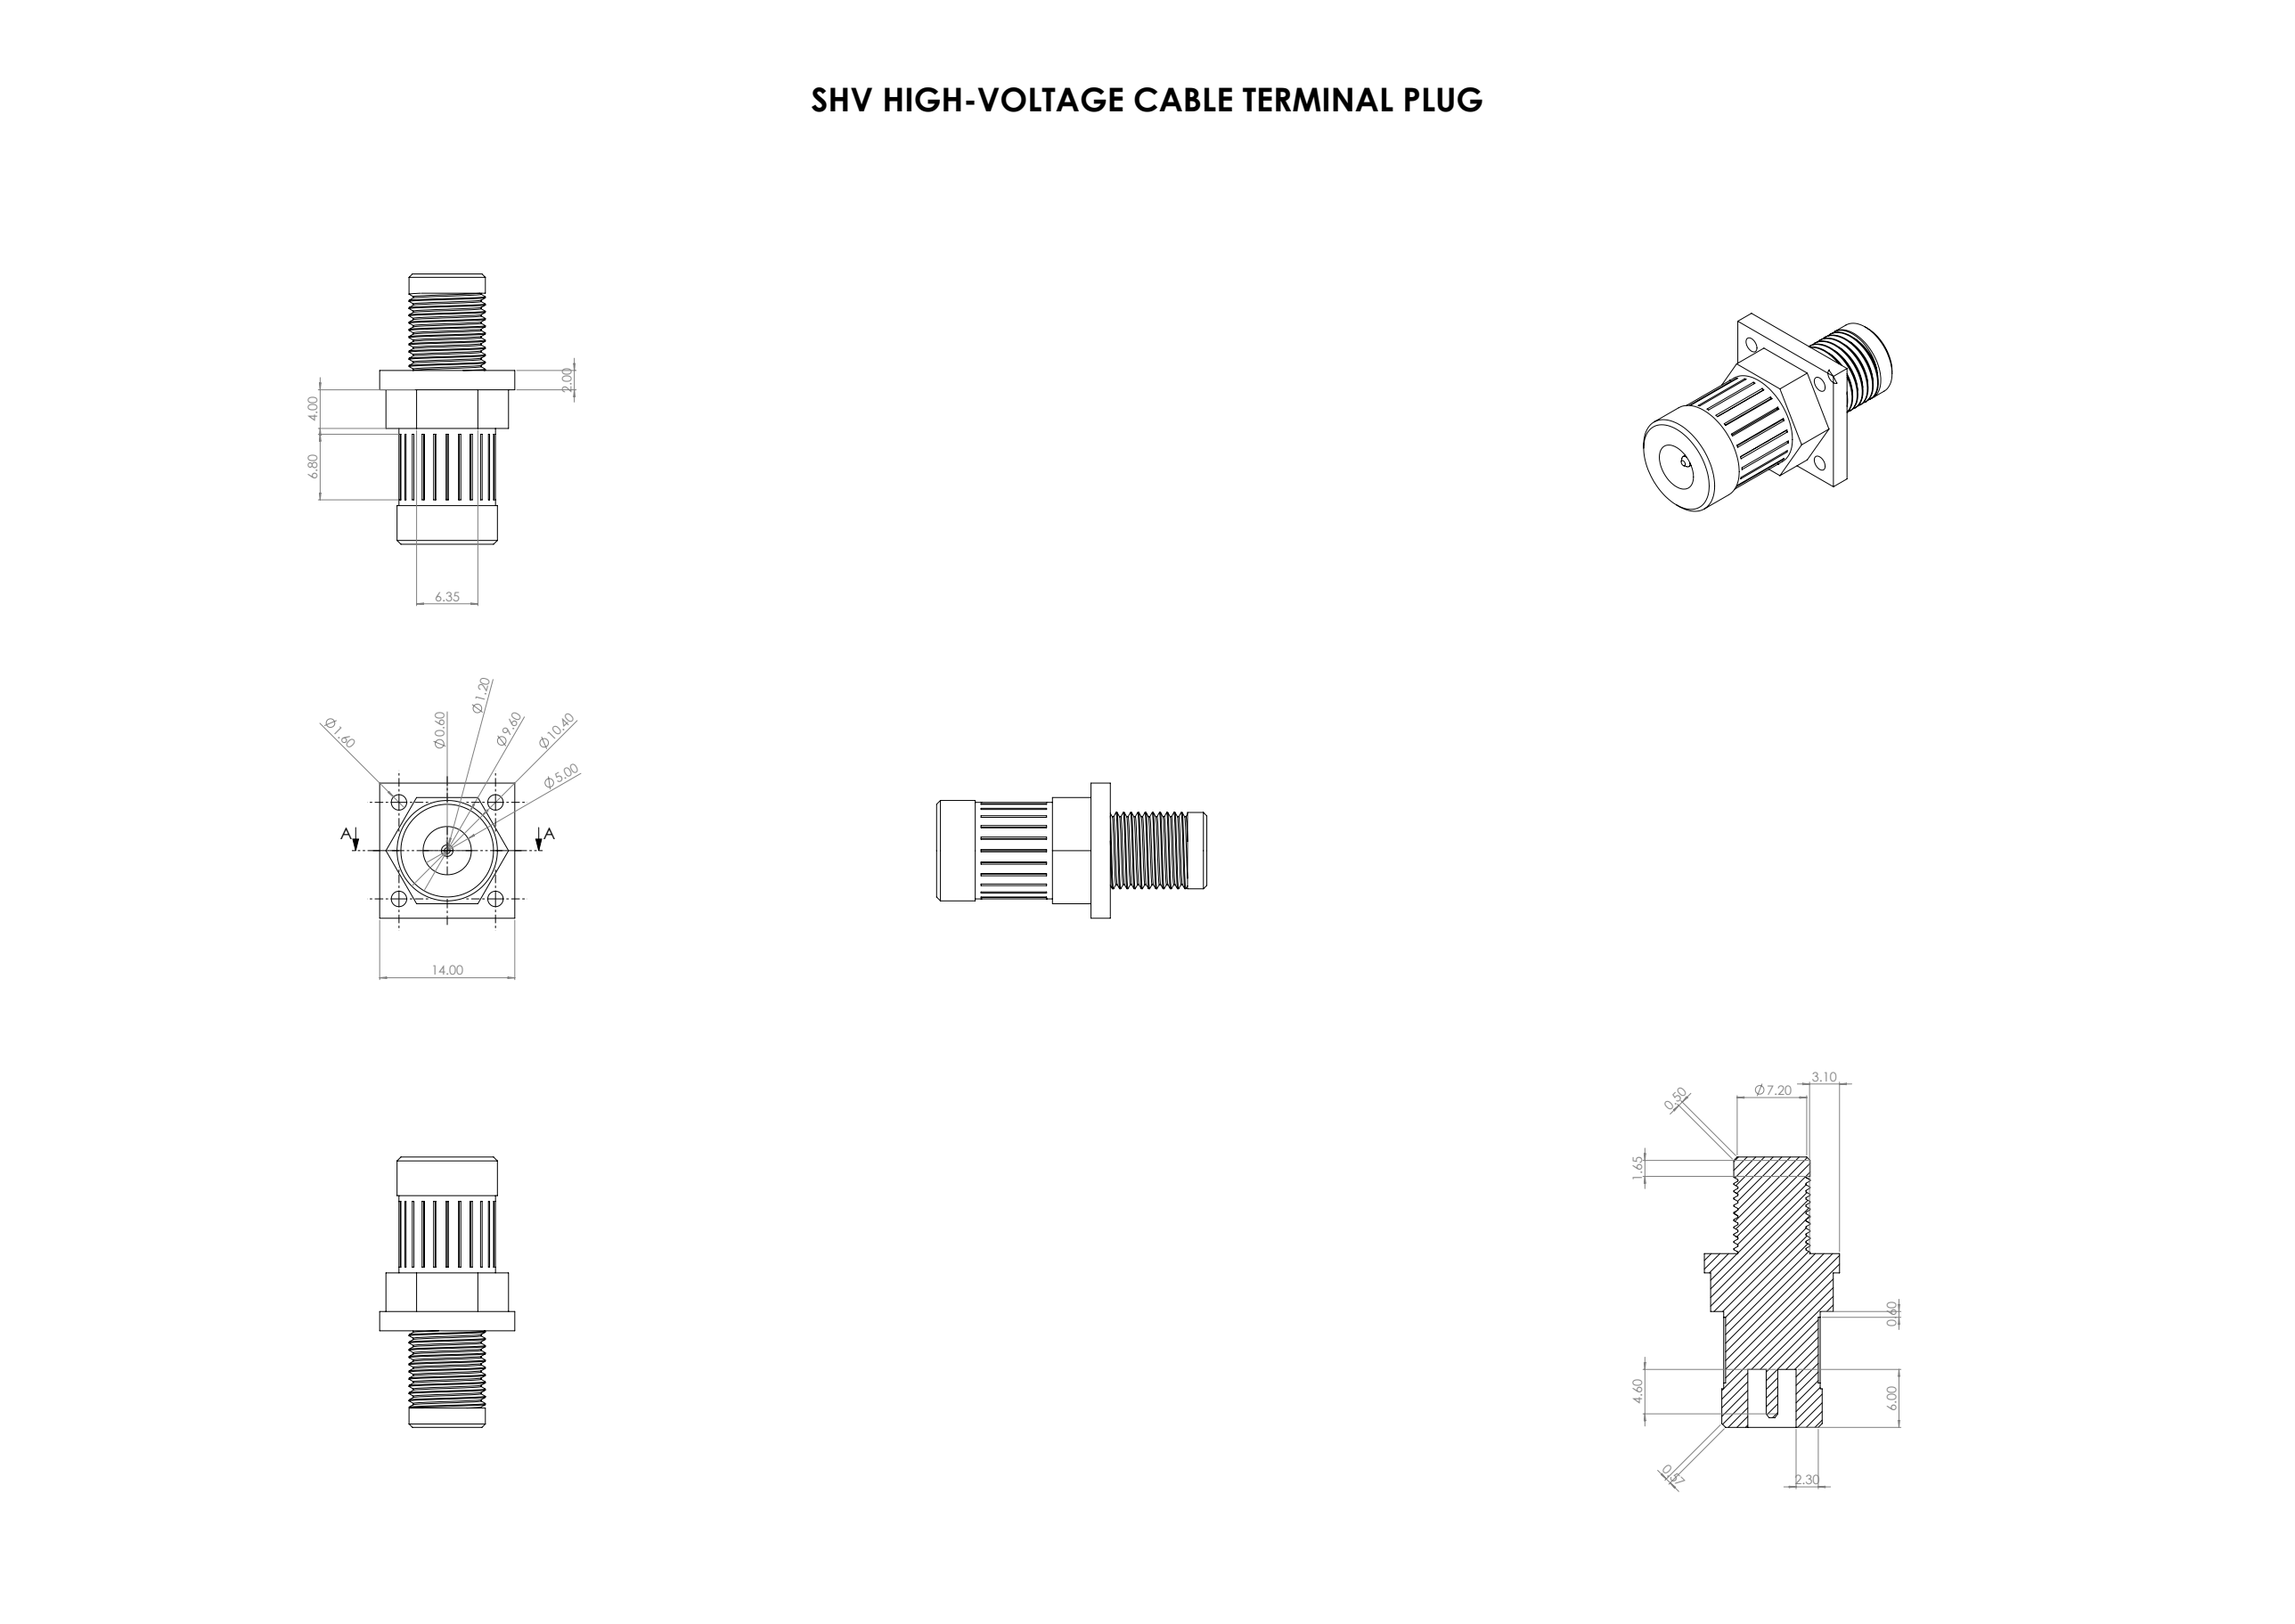
ISO-10303-21;
HEADER;
/* Generated by software containing ST-Developer
 * from STEP Tools, Inc. (www.steptools.com) 
 */

FILE_DESCRIPTION(
/* description */ (''),
/* implementation_level */ '2;1');

FILE_NAME(
/* name */ '13_SHV_High-Voltage_Cable_Terminal_Plug.step',
/* time_stamp */ '2026-10-19T22:59:19-07:00',
/* author */ (''),
/* organization */ (''),
/* preprocessor_version */ 'ST-DEVELOPER v20.2',
/* originating_system */ 'Autodesk Translation Framework v15.15.0.0',
/* authorisation */ '');

FILE_SCHEMA (('AUTOMOTIVE_DESIGN { 1 0 10303 214 3 1 1 }'));
ENDSEC;

DATA;
#10=MECHANICAL_DESIGN_GEOMETRIC_PRESENTATION_REPRESENTATION('',(#916),#53650);
#363=B_SPLINE_SURFACE_WITH_KNOTS('',3,3,((#34003,#34004,#34005,#34006,#34007,
#34008,#34009,#34010,#34011,#34012,#34013,#34014,#34015,#34016,#34017,#34018,
#34019,#34020,#34021,#34022,#34023,#34024,#34025,#34026,#34027,#34028,#34029,
#34030,#34031,#34032,#34033,#34034,#34035,#34036,#34037,#34038,#34039,#34040,
#34041,#34042,#34043,#34044,#34045,#34046,#34047,#34048,#34049,#34050,#34051,
#34052,#34053,#34054,#34055,#34056,#34057,#34058,#34059,#34060,#34061,#34062,
#34063,#34064,#34065,#34066,#34067,#34068,#34069,#34070,#34071,#34072,#34073,
#34074,#34075),(#34076,#34077,#34078,#34079,#34080,#34081,#34082,#34083,
#34084,#34085,#34086,#34087,#34088,#34089,#34090,#34091,#34092,#34093,#34094,
#34095,#34096,#34097,#34098,#34099,#34100,#34101,#34102,#34103,#34104,#34105,
#34106,#34107,#34108,#34109,#34110,#34111,#34112,#34113,#34114,#34115,#34116,
#34117,#34118,#34119,#34120,#34121,#34122,#34123,#34124,#34125,#34126,#34127,
#34128,#34129,#34130,#34131,#34132,#34133,#34134,#34135,#34136,#34137,#34138,
#34139,#34140,#34141,#34142,#34143,#34144,#34145,#34146,#34147,#34148),
(#34149,#34150,#34151,#34152,#34153,#34154,#34155,#34156,#34157,#34158,
#34159,#34160,#34161,#34162,#34163,#34164,#34165,#34166,#34167,#34168,#34169,
#34170,#34171,#34172,#34173,#34174,#34175,#34176,#34177,#34178,#34179,#34180,
#34181,#34182,#34183,#34184,#34185,#34186,#34187,#34188,#34189,#34190,#34191,
#34192,#34193,#34194,#34195,#34196,#34197,#34198,#34199,#34200,#34201,#34202,
#34203,#34204,#34205,#34206,#34207,#34208,#34209,#34210,#34211,#34212,#34213,
#34214,#34215,#34216,#34217,#34218,#34219,#34220,#34221),(#34222,#34223,
#34224,#34225,#34226,#34227,#34228,#34229,#34230,#34231,#34232,#34233,#34234,
#34235,#34236,#34237,#34238,#34239,#34240,#34241,#34242,#34243,#34244,#34245,
#34246,#34247,#34248,#34249,#34250,#34251,#34252,#34253,#34254,#34255,#34256,
#34257,#34258,#34259,#34260,#34261,#34262,#34263,#34264,#34265,#34266,#34267,
#34268,#34269,#34270,#34271,#34272,#34273,#34274,#34275,#34276,#34277,#34278,
#34279,#34280,#34281,#34282,#34283,#34284,#34285,#34286,#34287,#34288,#34289,
#34290,#34291,#34292,#34293,#34294)),.UNSPECIFIED.,.F.,.F.,.F.,(4,4),(4,
1,1,1,1,1,1,1,1,1,1,1,1,1,1,1,1,1,1,1,1,1,1,1,1,1,1,1,1,1,1,1,1,1,1,1,1,
1,1,1,1,1,1,1,1,1,1,1,1,1,1,1,1,1,1,1,1,1,1,1,1,1,1,1,1,1,1,1,1,1,4),(0.,
0.0496809906637673),(9.51827045652186,10.5054372529097,11.4926040492975,
12.4797708456853,13.4669376420731,14.4541044384609,15.4412712348487,16.4284380312366,
17.4156048276244,18.4027716240122,19.3899384204,20.3771052167878,21.3642720131756,
22.3514388095634,23.3386056059513,24.3257724023391,25.3129391987269,26.3001059951147,
27.2872727915025,28.2744395878903,29.2616063842781,30.2487731806659,31.2359399770538,
32.2231067734416,33.2102735698294,34.1974403662172,35.184607162605,36.1717739589928,
37.1589407553806,38.1461075517685,39.1332743481563,40.1204411445441,41.1076079409319,
42.0947747373197,43.0819415337075,44.0691083300953,45.0562751264832,46.043441922871,
47.0306087192588,48.0177755156466,49.0049423120344,49.9921091084222,50.97927590481,
51.9664427011978,52.9536094975857,53.9407762939735,54.9279430903613,55.9151098867491,
56.9022766831369,57.8894434795247,58.8766102759126,59.8637770723004,60.8509438686882,
61.838110665076,62.8252774614638,63.8124442578516,64.7996110542394,65.7867778506272,
66.7739446470151,67.7611114434029,68.7482782397907,69.7354450361785,70.7226118325663,
71.7097786289541,72.696945425342,73.6841122217298,74.6712790181176,75.6584458145054,
76.6456126108932,77.632779407281,78.6199462036688),.UNSPECIFIED.);
#364=B_SPLINE_SURFACE_WITH_KNOTS('',3,3,((#34517,#34518,#34519,#34520,#34521,
#34522,#34523,#34524,#34525,#34526,#34527,#34528,#34529,#34530,#34531,#34532,
#34533,#34534,#34535,#34536,#34537,#34538,#34539,#34540,#34541,#34542,#34543,
#34544,#34545,#34546,#34547,#34548,#34549,#34550,#34551,#34552,#34553,#34554,
#34555,#34556,#34557,#34558,#34559,#34560,#34561,#34562,#34563,#34564,#34565,
#34566,#34567,#34568,#34569,#34570,#34571,#34572,#34573,#34574,#34575,#34576,
#34577,#34578,#34579,#34580,#34581,#34582,#34583,#34584,#34585,#34586,#34587,
#34588,#34589),(#34590,#34591,#34592,#34593,#34594,#34595,#34596,#34597,
#34598,#34599,#34600,#34601,#34602,#34603,#34604,#34605,#34606,#34607,#34608,
#34609,#34610,#34611,#34612,#34613,#34614,#34615,#34616,#34617,#34618,#34619,
#34620,#34621,#34622,#34623,#34624,#34625,#34626,#34627,#34628,#34629,#34630,
#34631,#34632,#34633,#34634,#34635,#34636,#34637,#34638,#34639,#34640,#34641,
#34642,#34643,#34644,#34645,#34646,#34647,#34648,#34649,#34650,#34651,#34652,
#34653,#34654,#34655,#34656,#34657,#34658,#34659,#34660,#34661,#34662),
(#34663,#34664,#34665,#34666,#34667,#34668,#34669,#34670,#34671,#34672,
#34673,#34674,#34675,#34676,#34677,#34678,#34679,#34680,#34681,#34682,#34683,
#34684,#34685,#34686,#34687,#34688,#34689,#34690,#34691,#34692,#34693,#34694,
#34695,#34696,#34697,#34698,#34699,#34700,#34701,#34702,#34703,#34704,#34705,
#34706,#34707,#34708,#34709,#34710,#34711,#34712,#34713,#34714,#34715,#34716,
#34717,#34718,#34719,#34720,#34721,#34722,#34723,#34724,#34725,#34726,#34727,
#34728,#34729,#34730,#34731,#34732,#34733,#34734,#34735),(#34736,#34737,
#34738,#34739,#34740,#34741,#34742,#34743,#34744,#34745,#34746,#34747,#34748,
#34749,#34750,#34751,#34752,#34753,#34754,#34755,#34756,#34757,#34758,#34759,
#34760,#34761,#34762,#34763,#34764,#34765,#34766,#34767,#34768,#34769,#34770,
#34771,#34772,#34773,#34774,#34775,#34776,#34777,#34778,#34779,#34780,#34781,
#34782,#34783,#34784,#34785,#34786,#34787,#34788,#34789,#34790,#34791,#34792,
#34793,#34794,#34795,#34796,#34797,#34798,#34799,#34800,#34801,#34802,#34803,
#34804,#34805,#34806,#34807,#34808)),.UNSPECIFIED.,.F.,.F.,.F.,(4,4),(4,
1,1,1,1,1,1,1,1,1,1,1,1,1,1,1,1,1,1,1,1,1,1,1,1,1,1,1,1,1,1,1,1,1,1,1,1,
1,1,1,1,1,1,1,1,1,1,1,1,1,1,1,1,1,1,1,1,1,1,1,1,1,1,1,1,1,1,1,1,1,4),(0.,
0.0496809906637673),(12.8380991276371,13.8252659240249,14.8124327204127,
15.7995995168005,16.7867663131883,17.7739331095761,18.7610999059639,19.7482667023518,
20.7354334987396,21.7226002951274,22.7097670915152,23.696933887903,24.6841006842908,
25.6712674806786,26.6584342770665,27.6456010734543,28.6327678698421,29.6199346662299,
30.6071014626177,31.5942682590055,32.5814350553933,33.5686018517812,34.555768648169,
35.5429354445568,36.5301022409446,37.5172690373324,38.5044358337202,39.491602630108,
40.4787694264959,41.4659362228837,42.4531030192715,43.4402698156593,44.4274366120471,
45.4146034084349,46.4017702048227,47.3889370012105,48.3761037975984,49.3632705939862,
50.350437390374,51.3376041867618,52.3247709831496,53.3119377795374,54.2991045759252,
55.2862713723131,56.2734381687009,57.2606049650887,58.2477717614765,59.2349385578643,
60.2221053542521,61.2092721506399,62.1964389470278,63.1836057434156,64.1707725398034,
65.1579393361912,66.145106132579,67.1322729289668,68.1194397253546,69.1066065217424,
70.0937733181303,71.0809401145181,72.0681069109059,73.0552737072937,74.0424405036815,
75.0296073000693,76.0167740964572,77.003940892845,77.9911076892328,78.9782744856206,
79.9654412820084,80.9526080783962,81.939774874784),.UNSPECIFIED.);
#373=B_SPLINE_CURVE_WITH_KNOTS('',3,(#33239,#33240,#33241,#33242,#33243,
#33244,#33245,#33246,#33247,#33248,#33249,#33250,#33251,#33252,#33253,#33254,
#33255,#33256,#33257,#33258,#33259,#33260,#33261,#33262,#33263),
 .UNSPECIFIED.,.F.,.F.,(4,3,3,3,3,3,3,3,4),(-9.15304944749145,-8.88450116749033,
-7.89733437110252,-6.9101675747147,-5.92300077832689,-4.93583398193907,
-3.94866718555126,-2.96150038916344,-2.86986414031186),.UNSPECIFIED.);
#374=B_SPLINE_CURVE_WITH_KNOTS('',3,(#33268,#33269,#33270,#33271),
 .UNSPECIFIED.,.F.,.F.,(4,4),(-2.86986414031186,-2.08103247056473),
 .UNSPECIFIED.);
#375=B_SPLINE_CURVE_WITH_KNOTS('',3,(#33274,#33275,#33276,#33277,#33278,
#33279,#33280,#33281,#33282,#33283,#33284,#33285,#33286,#33287,#33288,#33289,
#33290,#33291,#33292,#33293,#33294,#33295),.UNSPECIFIED.,.F.,.F.,(4,3,3,
3,3,3,3,4),(0.,0.98716679638781,1.97433359277563,2.96150038916344,3.94866718555125,
4.93583398193907,5.92300077832688,6.18969281142703),.UNSPECIFIED.);
#376=B_SPLINE_CURVE_WITH_KNOTS('',3,(#33300,#33301,#33302,#33303,#33304,
#33305,#33306,#33307,#33308,#33309,#33310,#33311,#33312,#33313,#33314,#33315,
#33316,#33317,#33318,#33319,#33320,#33321),.UNSPECIFIED.,.F.,.F.,(4,3,3,
3,3,3,3,4),(-15.436234754671,-14.8075019458172,-13.8203351494294,-12.8331683530416,
-11.8460015566538,-10.858834760266,-9.87166796387814,-9.15304944749145),
 .UNSPECIFIED.);
#377=B_SPLINE_CURVE_WITH_KNOTS('',3,(#33322,#33323,#33324,#33325,#33326,
#33327,#33328,#33329,#33330,#33331,#33332,#33333,#33334,#33335,#33336,#33337,
#33338,#33339,#33340,#33341,#33342,#33343),.UNSPECIFIED.,.F.,.F.,(4,3,3,
3,3,3,3,4),(6.18969281142703,6.9101675747147,7.89733437110251,8.88450116749032,
9.87166796387814,10.858834760266,11.8460015566538,12.4728781186066),
 .UNSPECIFIED.);
#378=B_SPLINE_CURVE_WITH_KNOTS('',3,(#33348,#33349,#33350,#33351,#33352,
#33353,#33354,#33355,#33356,#33357,#33358,#33359,#33360,#33361,#33362,#33363,
#33364,#33365,#33366,#33367,#33368,#33369),.UNSPECIFIED.,.F.,.F.,(4,3,3,
3,3,3,3,4),(-21.7194200618506,-20.7305027241441,-19.7433359277563,-18.7561691313685,
-17.7690023349807,-16.7818355385928,-15.794668742205,-15.436234754671),
 .UNSPECIFIED.);
#379=B_SPLINE_CURVE_WITH_KNOTS('',3,(#33370,#33371,#33372,#33373,#33374,
#33375,#33376,#33377,#33378,#33379,#33380,#33381,#33382,#33383,#33384,#33385,
#33386,#33387,#33388,#33389,#33390,#33391),.UNSPECIFIED.,.F.,.F.,(4,3,3,
3,3,3,3,4),(12.4728781186066,12.8331683530416,13.8203351494294,14.8075019458172,
15.794668742205,16.7818355385928,17.7690023349807,18.7560634257862),
 .UNSPECIFIED.);
#380=B_SPLINE_CURVE_WITH_KNOTS('',3,(#33396,#33397,#33398,#33399,#33400,
#33401,#33402,#33403,#33404,#33405,#33406,#33407,#33408,#33409,#33410,#33411,
#33412,#33413,#33414,#33415,#33416,#33417),.UNSPECIFIED.,.F.,.F.,(4,3,3,
3,3,3,3,4),(-28.0026053690302,-27.6406702988588,-26.653503502471,-25.6663367060832,
-24.6791699096953,-23.6920031133075,-22.7048363169197,-21.7194200618506),
 .UNSPECIFIED.);
#381=B_SPLINE_CURVE_WITH_KNOTS('',3,(#33418,#33419,#33420,#33421,#33422,
#33423,#33424,#33425,#33426,#33427,#33428,#33429,#33430,#33431,#33432,#33433,
#33434,#33435,#33436,#33437,#33438,#33439),.UNSPECIFIED.,.F.,.F.,(4,3,3,
3,3,3,3,4),(18.7560634257862,19.7433359277563,20.7305027241441,21.7176695205319,
22.7048363169197,23.6920031133075,24.6791699096954,25.0392487329658),
 .UNSPECIFIED.);
#382=B_SPLINE_CURVE_WITH_KNOTS('',3,(#33444,#33445,#33446,#33447,#33448,
#33449,#33450,#33451,#33452,#33453,#33454,#33455,#33456,#33457,#33458,#33459,
#33460,#33461,#33462,#33463,#33464,#33465),.UNSPECIFIED.,.F.,.F.,(4,3,3,
3,3,3,3,4),(-34.2857906762098,-33.5636710771857,-32.5765042807979,-31.58933748441,
-30.6021706880222,-29.6150038916344,-28.6278370952466,-28.0026053690302),
 .UNSPECIFIED.);
#383=B_SPLINE_CURVE_WITH_KNOTS('',3,(#33466,#33467,#33468,#33469,#33470,
#33471,#33472,#33473,#33474,#33475,#33476,#33477,#33478,#33479,#33480,#33481,
#33482,#33483,#33484,#33485,#33486,#33487),.UNSPECIFIED.,.F.,.F.,(4,3,3,
3,3,3,3,4),(25.0392487329658,25.6663367060832,26.653503502471,27.6406702988588,
28.6278370952466,29.6150038916344,30.6021706880222,31.3224340401454),
 .UNSPECIFIED.);
#384=B_SPLINE_CURVE_WITH_KNOTS('',3,(#33492,#33493,#33494,#33495,#33496,
#33497,#33498,#33499,#33500,#33501,#33502,#33503,#33504,#33505,#33506,#33507,
#33508,#33509,#33510,#33511,#33512,#33513,#33514,#33515,#33516),
 .UNSPECIFIED.,.F.,.F.,(4,3,3,3,3,3,3,3,4),(-40.5689759833894,-40.4738386519004,
-39.4866718555126,-38.4995050591247,-37.5123382627369,-36.5251714663491,
-35.5380046699613,-34.5508378735735,-34.2857906762098),.UNSPECIFIED.);
#385=B_SPLINE_CURVE_WITH_KNOTS('',3,(#33517,#33518,#33519,#33520,#33521,
#33522,#33523,#33524,#33525,#33526,#33527,#33528,#33529,#33530,#33531,#33532,
#33533,#33534,#33535,#33536,#33537,#33538,#33539,#33540,#33541),
 .UNSPECIFIED.,.F.,.F.,(4,3,3,3,3,3,3,3,4),(31.3224340401454,31.58933748441,
32.5765042807979,33.5636710771857,34.5508378735735,35.5380046699613,36.5251714663491,
37.5123382627369,37.605619347325),.UNSPECIFIED.);
#386=B_SPLINE_CURVE_WITH_KNOTS('',3,(#33546,#33547,#33548,#33549,#33550,
#33551,#33552,#33553,#33554,#33555,#33556,#33557,#33558,#33559,#33560,#33561,
#33562,#33563,#33564,#33565,#33566,#33567),.UNSPECIFIED.,.F.,.F.,(4,3,3,
3,3,3,3,4),(-46.852161290569,-46.3968394302273,-45.4096726338394,-44.4225058374516,
-43.4353390410638,-42.448172244676,-41.4610054482882,-40.5689759833894),
 .UNSPECIFIED.);
#387=B_SPLINE_CURVE_WITH_KNOTS('',3,(#33568,#33569,#33570,#33571,#33572,
#33573,#33574,#33575,#33576,#33577,#33578,#33579,#33580,#33581,#33582,#33583,
#33584,#33585,#33586,#33587,#33588,#33589),.UNSPECIFIED.,.F.,.F.,(4,3,3,
3,3,3,3,4),(37.605619347325,38.4995050591248,39.4866718555126,40.4738386519004,
41.4610054482882,42.448172244676,43.4353390410638,43.8888046545046),
 .UNSPECIFIED.);
#388=B_SPLINE_CURVE_WITH_KNOTS('',3,(#33594,#33595,#33596,#33597,#33598,
#33599,#33600,#33601,#33602,#33603,#33604,#33605,#33606,#33607,#33608,#33609,
#33610,#33611,#33612,#33613,#33614,#33615),.UNSPECIFIED.,.F.,.F.,(4,3,3,
3,3,3,3,4),(-53.1353465977486,-52.3198402085541,-51.3326734121663,-50.3455066157785,
-49.3583398193907,-48.3711730230029,-47.3840062266151,-46.852161290569),
 .UNSPECIFIED.);
#389=B_SPLINE_CURVE_WITH_KNOTS('',3,(#33616,#33617,#33618,#33619,#33620,
#33621,#33622,#33623,#33624,#33625,#33626,#33627,#33628,#33629,#33630,#33631,
#33632,#33633,#33634,#33635,#33636,#33637),.UNSPECIFIED.,.F.,.F.,(4,3,3,
3,3,3,3,4),(43.8888046545046,44.4225058374516,45.4096726338394,46.3968394302273,
47.3840062266151,48.3711730230029,49.3583398193907,50.1719899616841),
 .UNSPECIFIED.);
#390=B_SPLINE_CURVE_WITH_KNOTS('',3,(#33642,#33643,#33644,#33645,#33646,
#33647,#33648,#33649,#33650,#33651,#33652,#33653,#33654,#33655,#33656,#33657,
#33658,#33659,#33660,#33661,#33662,#33663,#33664,#33665,#33666),
 .UNSPECIFIED.,.F.,.F.,(4,3,3,3,3,3,3,3,4),(-59.4185319049282,-59.2300077832689,
-58.242840986881,-57.2556741904932,-56.2685073941054,-55.2813405977176,
-54.2941738013298,-53.307007004942,-53.1353465977486),.UNSPECIFIED.);
#391=B_SPLINE_CURVE_WITH_KNOTS('',3,(#33667,#33668,#33669,#33670,#33671,
#33672,#33673,#33674,#33675,#33676,#33677,#33678,#33679,#33680,#33681,#33682,
#33683,#33684,#33685,#33686,#33687,#33688,#33689,#33690,#33691),
 .UNSPECIFIED.,.F.,.F.,(4,3,3,3,3,3,3,3,4),(50.1719899616841,50.3455066157785,
51.3326734121663,52.3198402085541,53.307007004942,54.2941738013298,55.2813405977176,
56.2685073941054,56.4551752688637),.UNSPECIFIED.);
#392=B_SPLINE_CURVE_WITH_KNOTS('',3,(#33696,#33697,#33698,#33699,#33700,
#33701,#33702,#33703,#33704,#33705,#33706,#33707,#33708,#33709,#33710,#33711,
#33712,#33713,#33714,#33715,#33716,#33717),.UNSPECIFIED.,.F.,.F.,(4,3,3,
3,3,3,3,4),(-65.7017172121077,-65.1530085615957,-64.1658417652079,-63.1786749688201,
-62.1915081724323,-61.2043413760445,-60.2171745796567,-59.4185319049282),
 .UNSPECIFIED.);
#393=B_SPLINE_CURVE_WITH_KNOTS('',3,(#33718,#33719,#33720,#33721,#33722,
#33723,#33724,#33725,#33726,#33727,#33728,#33729,#33730,#33731,#33732,#33733,
#33734,#33735,#33736,#33737,#33738,#33739),.UNSPECIFIED.,.F.,.F.,(4,3,3,
3,3,3,3,4),(56.4551752688637,57.2556741904932,58.242840986881,59.2300077832688,
60.2171745796566,61.2043413760445,62.1915081724323,62.7383605760433),
 .UNSPECIFIED.);
#394=B_SPLINE_CURVE_WITH_KNOTS('',3,(#33745,#33746,#33747,#33748,#33749),
 .UNSPECIFIED.,.F.,.F.,(4,1,4),(78.5398163397448,78.9782744856206,79.8587424042193),
 .UNSPECIFIED.);
#395=B_SPLINE_CURVE_WITH_KNOTS('',3,(#33752,#33753,#33754,#33755),
 .UNSPECIFIED.,.F.,.F.,(4,4),(78.5398163397448,78.6199462036688),
 .UNSPECIFIED.);
#396=B_SPLINE_CURVE_WITH_KNOTS('',3,(#33760,#33761,#33762,#33763,#33764,
#33765,#33766,#33767,#33768,#33769),.UNSPECIFIED.,.F.,.F.,(4,1,1,1,1,1,
1,4),(72.2566310325652,73.0552737072937,74.0424405036815,75.0296073000693,
76.0167740964572,77.003940892845,77.9911076892328,78.5398163397448),
 .UNSPECIFIED.);
#397=B_SPLINE_CURVE_WITH_KNOTS('',3,(#33770,#33771,#33772,#33773,#33774,
#33775,#33776,#33777,#33778,#33779),.UNSPECIFIED.,.F.,.F.,(4,1,1,1,1,1,
1,4),(72.2566310325652,72.696945425342,73.6841122217298,74.6712790181176,
75.6584458145054,76.6456126108932,77.632779407281,78.5398163397448),
 .UNSPECIFIED.);
#398=B_SPLINE_CURVE_WITH_KNOTS('',3,(#33784,#33785,#33786,#33787,#33788,
#33789,#33790,#33791,#33792,#33793,#33794),.UNSPECIFIED.,.F.,.F.,(4,1,1,
1,1,1,1,1,4),(65.9734457253856,66.145106132579,67.1322729289668,68.1194397253546,
69.1066065217424,70.0937733181303,71.0809401145181,72.0681069109059,72.2566310325652),
 .UNSPECIFIED.);
#399=B_SPLINE_CURVE_WITH_KNOTS('',3,(#33795,#33796,#33797,#33798,#33799,
#33800,#33801,#33802,#33803,#33804),.UNSPECIFIED.,.F.,.F.,(4,1,1,1,1,1,
1,4),(65.9734457253856,66.7739446470151,67.7611114434029,68.7482782397907,
69.7354450361785,70.7226118325663,71.7097786289541,72.2566310325652),
 .UNSPECIFIED.);
#400=B_SPLINE_CURVE_WITH_KNOTS('',3,(#33809,#33810,#33811,#33812,#33813,
#33814,#33815,#33816,#33817,#33818),.UNSPECIFIED.,.F.,.F.,(4,1,1,1,1,1,
1,4),(59.6902604182061,60.2221053542521,61.2092721506399,62.1964389470278,
63.1836057434156,64.1707725398034,65.1579393361912,65.9734457253856),
 .UNSPECIFIED.);
#401=B_SPLINE_CURVE_WITH_KNOTS('',3,(#33819,#33820,#33821,#33822,#33823,
#33824,#33825,#33826,#33827,#33828,#33829),.UNSPECIFIED.,.F.,.F.,(4,1,1,
1,1,1,1,1,4),(59.6902604182061,59.8637770723004,60.8509438686882,61.838110665076,
62.8252774614638,63.8124442578516,64.7996110542394,65.7867778506272,65.9734457253856),
 .UNSPECIFIED.);
#402=B_SPLINE_CURVE_WITH_KNOTS('',3,(#33834,#33835,#33836,#33837,#33838,
#33839,#33840,#33841,#33842,#33843),.UNSPECIFIED.,.F.,.F.,(4,1,1,1,1,1,
1,4),(53.4070751110265,54.2991045759252,55.2862713723131,56.2734381687009,
57.2606049650887,58.2477717614765,59.2349385578643,59.6902604182061),
 .UNSPECIFIED.);
#403=B_SPLINE_CURVE_WITH_KNOTS('',3,(#33844,#33845,#33846,#33847,#33848,
#33849,#33850,#33851,#33852,#33853),.UNSPECIFIED.,.F.,.F.,(4,1,1,1,1,1,
1,4),(53.4070751110265,53.9407762939735,54.9279430903613,55.9151098867491,
56.9022766831369,57.8894434795247,58.8766102759126,59.6902604182061),
 .UNSPECIFIED.);
#404=B_SPLINE_CURVE_WITH_KNOTS('',3,(#33858,#33859,#33860,#33861,#33862,
#33863,#33864,#33865,#33866,#33867,#33868),.UNSPECIFIED.,.F.,.F.,(4,1,1,
1,1,1,1,1,4),(47.1238898038469,47.3889370012105,48.3761037975984,49.3632705939862,
50.350437390374,51.3376041867618,52.3247709831496,53.3119377795374,53.4070751110265),
 .UNSPECIFIED.);
#405=B_SPLINE_CURVE_WITH_KNOTS('',3,(#33869,#33870,#33871,#33872,#33873,
#33874,#33875,#33876,#33877,#33878),.UNSPECIFIED.,.F.,.F.,(4,1,1,1,1,1,
1,4),(47.1238898038469,48.0177755156466,49.0049423120344,49.9921091084222,
50.97927590481,51.9664427011978,52.9536094975857,53.4070751110265),
 .UNSPECIFIED.);
#406=B_SPLINE_CURVE_WITH_KNOTS('',3,(#33883,#33884,#33885,#33886,#33887,
#33888,#33889,#33890,#33891,#33892),.UNSPECIFIED.,.F.,.F.,(4,1,1,1,1,1,
1,4),(40.8407044966673,41.4659362228837,42.4531030192715,43.4402698156593,
44.4274366120471,45.4146034084349,46.4017702048227,47.1238898038469),
 .UNSPECIFIED.);
#407=B_SPLINE_CURVE_WITH_KNOTS('',3,(#33893,#33894,#33895,#33896,#33897,
#33898,#33899,#33900,#33901,#33902,#33903),.UNSPECIFIED.,.F.,.F.,(4,1,1,
1,1,1,1,1,4),(40.8407044966673,41.1076079409319,42.0947747373197,43.0819415337075,
44.0691083300953,45.0562751264832,46.043441922871,47.0306087192588,47.1238898038469),
 .UNSPECIFIED.);
#408=B_SPLINE_CURVE_WITH_KNOTS('',3,(#33908,#33909,#33910,#33911,#33912,
#33913,#33914,#33915,#33916,#33917),.UNSPECIFIED.,.F.,.F.,(4,1,1,1,1,1,
1,4),(34.5575191894877,35.5429354445568,36.5301022409446,37.5172690373324,
38.5044358337202,39.491602630108,40.4787694264959,40.8407044966673),
 .UNSPECIFIED.);
#409=B_SPLINE_CURVE_WITH_KNOTS('',3,(#33918,#33919,#33920,#33921,#33922,
#33923,#33924,#33925,#33926,#33927),.UNSPECIFIED.,.F.,.F.,(4,1,1,1,1,1,
1,4),(34.5575191894877,35.184607162605,36.1717739589928,37.1589407553806,
38.1461075517685,39.1332743481563,40.1204411445441,40.8407044966673),
 .UNSPECIFIED.);
#410=B_SPLINE_CURVE_WITH_KNOTS('',3,(#33932,#33933,#33934,#33935,#33936,
#33937,#33938,#33939,#33940,#33941,#33942),.UNSPECIFIED.,.F.,.F.,(4,1,1,
1,1,1,1,1,4),(28.2743338823081,28.6327678698421,29.6199346662299,30.6071014626177,
31.5942682590055,32.5814350553933,33.5686018517812,34.555768648169,34.5575191894877),
 .UNSPECIFIED.);
#411=B_SPLINE_CURVE_WITH_KNOTS('',3,(#33943,#33944,#33945,#33946,#33947,
#33948,#33949,#33950,#33951,#33952,#33953),.UNSPECIFIED.,.F.,.F.,(4,1,1,
1,1,1,1,1,4),(28.2743338823081,28.2744395878903,29.2616063842781,30.2487731806659,
31.2359399770538,32.2231067734416,33.2102735698294,34.1974403662172,34.5575191894877),
 .UNSPECIFIED.);
#412=B_SPLINE_CURVE_WITH_KNOTS('',3,(#33958,#33959,#33960,#33961,#33962,
#33963,#33964,#33965,#33966,#33967),.UNSPECIFIED.,.F.,.F.,(4,1,1,1,1,1,
1,4),(21.9911485751285,22.7097670915152,23.696933887903,24.6841006842908,
25.6712674806786,26.6584342770665,27.6456010734543,28.2743338823081),
 .UNSPECIFIED.);
#413=B_SPLINE_CURVE_WITH_KNOTS('',3,(#33968,#33969,#33970,#33971,#33972,
#33973,#33974,#33975,#33976,#33977),.UNSPECIFIED.,.F.,.F.,(4,1,1,1,1,1,
1,4),(21.9911485751285,22.3514388095634,23.3386056059513,24.3257724023391,
25.3129391987269,26.3001059951147,27.2872727915025,28.2743338823081),
 .UNSPECIFIED.);
#414=B_SPLINE_CURVE_WITH_KNOTS('',3,(#33982,#33983,#33984,#33985,#33986,
#33987,#33988,#33989,#33990,#33991,#33992),.UNSPECIFIED.,.F.,.F.,(4,1,1,
1,1,1,1,1,4),(15.7079632679489,15.7995995168005,16.7867663131883,17.7739331095761,
18.7610999059639,19.7482667023518,20.7354334987396,21.7226002951274,21.9911485751285),
 .UNSPECIFIED.);
#415=B_SPLINE_CURVE_WITH_KNOTS('',3,(#33993,#33994,#33995,#33996,#33997,
#33998,#33999,#34000,#34001,#34002),.UNSPECIFIED.,.F.,.F.,(4,1,1,1,1,1,
1,4),(15.7079632679489,16.4284380312366,17.4156048276244,18.4027716240122,
19.3899384204,20.3771052167878,21.3642720131756,21.9911485751285),
 .UNSPECIFIED.);
#416=B_SPLINE_CURVE_WITH_KNOTS('',3,(#34296,#34297,#34298,#34299,#34300,
#34301,#34302,#34303,#34304,#34305,#34306,#34307,#34308,#34309,#34310,#34311,
#34312,#34313,#34314,#34315,#34316,#34317,#34318,#34319,#34320,#34321,#34322,
#34323,#34324,#34325,#34326,#34327,#34328,#34329,#34330,#34331,#34332,#34333,
#34334,#34335,#34336,#34337,#34338,#34339,#34340,#34341,#34342,#34343,#34344,
#34345,#34346,#34347,#34348,#34349,#34350,#34351,#34352,#34353,#34354,#34355,
#34356),.UNSPECIFIED.,.F.,.F.,(4,3,3,3,3,3,3,3,3,3,3,3,3,3,3,3,3,3,3,3,
4),(-0.780432929098612,-0.738338012777856,-0.683834258573259,-0.663838565476387,
-0.598169338795401,-0.577510604236597,-0.562119826273733,-0.497408932506566,
-0.451782302166264,-0.430327346583771,-0.415002532446257,-0.359442543267042,
-0.314512225358661,-0.29120578257896,-0.270249996878916,-0.207616527572625,
-0.155712395679469,-0.140396343062156,-0.123829552848863,-0.0619147764244314,
0.),.UNSPECIFIED.);
#417=B_SPLINE_CURVE_WITH_KNOTS('',3,(#34357,#34358,#34359,#34360,#34361,
#34362,#34363,#34364,#34365,#34366,#34367,#34368,#34369,#34370,#34371,#34372),
 .UNSPECIFIED.,.F.,.F.,(4,3,3,3,3,4),(62.7383605760433,63.1786749688201,
64.1658417652079,65.1530085615957,66.1401753579835,67.0206432765822),
 .UNSPECIFIED.);
#418=B_SPLINE_CURVE_WITH_KNOTS('',3,(#34374,#34375,#34376,#34377,#34378,
#34379,#34380,#34381,#34382,#34383,#34384,#34385,#34386,#34387,#34388,#34389,
#34390,#34391,#34392,#34393,#34394,#34395,#34396,#34397,#34398,#34399,#34400,
#34401,#34402,#34403,#34404,#34405,#34406,#34407,#34408,#34409,#34410,#34411,
#34412,#34413,#34414,#34415,#34416,#34417,#34418,#34419,#34420,#34421,#34422,
#34423,#34424,#34425,#34426,#34427,#34428,#34429,#34430,#34431,#34432,#34433,
#34434,#34435,#34436,#34437),.UNSPECIFIED.,.F.,.F.,(4,3,3,3,3,3,3,3,3,3,
3,3,3,3,3,3,3,3,3,3,3,4),(-0.782320427274649,-0.744412510134687,-0.688529792301629,
-0.669642910660232,-0.618424444943536,-0.597739729117171,-0.580869545572353,
-0.517475334412603,-0.472408188284826,-0.451438075940233,-0.43660958913821,
-0.382241417220766,-0.33446124006817,-0.310889038365519,-0.29130300268306,
-0.227103495746363,-0.170327621809772,-0.152876921934579,-0.137524083313296,
-0.0687620416566481,-0.00415757966036404,0.),.UNSPECIFIED.);
#419=B_SPLINE_CURVE_WITH_KNOTS('',3,(#34438,#34439,#34440,#34441,#34442,
#34443,#34444,#34445),.UNSPECIFIED.,.F.,.F.,(4,1,1,1,1,4),(11.5993029270866,
12.4797708456853,13.4669376420731,14.4541044384609,15.4412712348487,15.7079632679489),
 .UNSPECIFIED.);
#420=B_SPLINE_CURVE_WITH_KNOTS('',3,(#34448,#34449,#34450,#34451,#34452,
#34453,#34454,#34455,#34456,#34457,#34458,#34459,#34460,#34461,#34462,#34463,
#34464,#34465,#34466,#34467,#34468,#34469,#34470,#34471,#34472,#34473,#34474,
#34475,#34476,#34477,#34478,#34479,#34480,#34481,#34482,#34483,#34484,#34485,
#34486,#34487,#34488,#34489,#34490,#34491,#34492,#34493,#34494,#34495,#34496,
#34497,#34498,#34499,#34500,#34501,#34502,#34503,#34504,#34505,#34506,#34507,
#34508),.UNSPECIFIED.,.F.,.F.,(4,3,3,3,3,3,3,3,3,3,3,3,3,3,3,3,3,3,3,3,
4),(-0.780432929098611,-0.738338012777859,-0.683834237462397,-0.663838555047122,
-0.598169328522835,-0.577510488075,-0.562119617951329,-0.497408718040529,
-0.45178193717698,-0.430324802159164,-0.415000406365485,-0.359442543267047,
-0.314512225358666,-0.29120578372101,-0.27024999961834,-0.207616508984274,
-0.155712381738205,-0.140396296964378,-0.123829546509967,-0.0619147732549836,
0.),.UNSPECIFIED.);
#421=B_SPLINE_CURVE_WITH_KNOTS('',3,(#34511,#34512,#34513,#34514,#34515,
#34516),.UNSPECIFIED.,.F.,.F.,(4,1,1,4),(12.8380991276371,13.8252659240249,
14.8124327204127,15.7079632679489),.UNSPECIFIED.);
#422=B_SPLINE_CURVE_WITH_KNOTS('',3,(#34810,#34811,#34812,#34813,#34814,
#34815,#34816,#34817,#34818,#34819,#34820,#34821,#34822,#34823,#34824,#34825,
#34826,#34827,#34828,#34829,#34830,#34831,#34832,#34833,#34834,#34835,#34836,
#34837,#34838,#34839,#34840,#34841,#34842,#34843,#34844,#34845,#34846,#34847,
#34848,#34849,#34850,#34851,#34852,#34853,#34854,#34855,#34856,#34857,#34858,
#34859,#34860,#34861,#34862,#34863,#34864,#34865,#34866,#34867,#34868,#34869,
#34870,#34871,#34872,#34873),.UNSPECIFIED.,.F.,.F.,(4,3,3,3,3,3,3,3,3,3,
3,3,3,3,3,3,3,3,3,3,3,4),(-0.782320427274647,-0.744412510134681,-0.688529784827506,
-0.669642900569953,-0.618424486060736,-0.597739627606828,-0.580869476506375,
-0.5174752643267,-0.472408127669552,-0.451437419639239,-0.436608276654843,
-0.38224141722077,-0.334461240068174,-0.310889049141467,-0.291303007297222,
-0.227103471436237,-0.170327603577178,-0.152876814667526,-0.137524066743929,
-0.0687620333719644,-0.00415763970634024,0.),.UNSPECIFIED.);
#423=B_SPLINE_CURVE_WITH_KNOTS('',3,(#34874,#34875,#34876,#34877,#34878,
#34879,#34880,#34881,#34882,#34883,#34884,#34885,#34886),.UNSPECIFIED.,
 .F.,.F.,(4,3,3,3,4),(-69.101675747147,-68.1145089507592,-67.1273421543714,
-66.1401753579836,-65.7017172121077),.UNSPECIFIED.);
#884=SHAPE_REPRESENTATION_RELATIONSHIP('SRR','None',#53729,#900);
#900=ADVANCED_BREP_SHAPE_REPRESENTATION('',(#932),#53639);
#916=STYLED_ITEM('',(#53972),#932);
#932=MANIFOLD_SOLID_BREP('SHV Plug',#23308);
#1000=CYLINDRICAL_SURFACE('',#24108,0.3954);
#1001=CYLINDRICAL_SURFACE('',#24111,0.3954);
#1002=CYLINDRICAL_SURFACE('',#24112,0.3954);
#1003=CYLINDRICAL_SURFACE('',#24113,0.3954);
#1004=CYLINDRICAL_SURFACE('',#24114,0.3954);
#1005=CYLINDRICAL_SURFACE('',#24115,0.3954);
#1006=CYLINDRICAL_SURFACE('',#24116,0.3954);
#1007=CYLINDRICAL_SURFACE('',#24117,0.3954);
#1008=CYLINDRICAL_SURFACE('',#24118,0.3954);
#1009=CYLINDRICAL_SURFACE('',#24119,0.3954);
#1010=CYLINDRICAL_SURFACE('',#24120,0.352375);
#1011=CYLINDRICAL_SURFACE('',#24122,0.352375);
#1012=CYLINDRICAL_SURFACE('',#24123,0.352375);
#1013=CYLINDRICAL_SURFACE('',#24124,0.352375);
#1014=CYLINDRICAL_SURFACE('',#24125,0.352375);
#1015=CYLINDRICAL_SURFACE('',#24126,0.352375);
#1016=CYLINDRICAL_SURFACE('',#24127,0.352375);
#1017=CYLINDRICAL_SURFACE('',#24128,0.352375);
#1018=CYLINDRICAL_SURFACE('',#24129,0.352375);
#1019=CYLINDRICAL_SURFACE('',#24130,0.352375);
#1020=CYLINDRICAL_SURFACE('',#24131,0.352375);
#1021=CYLINDRICAL_SURFACE('',#24134,0.352375);
#1022=CYLINDRICAL_SURFACE('',#24135,0.08);
#1023=CYLINDRICAL_SURFACE('',#24138,0.08);
#1024=CYLINDRICAL_SURFACE('',#24141,0.08);
#1025=CYLINDRICAL_SURFACE('',#24144,0.08);
#1026=CYLINDRICAL_SURFACE('',#24293,0.06);
#1027=CYLINDRICAL_SURFACE('',#24301,0.25);
#1028=CYLINDRICAL_SURFACE('',#24303,0.5);
#1029=CYLINDRICAL_SURFACE('',#24308,0.52);
#1030=CYLINDRICAL_SURFACE('',#24330,0.3954);
#1345=FACE_BOUND('',#4080,.T.);
#1346=FACE_BOUND('',#4083,.T.);
#1347=FACE_BOUND('',#4084,.T.);
#1348=FACE_BOUND('',#4085,.T.);
#1349=FACE_BOUND('',#4086,.T.);
#1350=FACE_BOUND('',#4087,.T.);
#1351=FACE_BOUND('',#4088,.T.);
#1352=FACE_BOUND('',#4089,.T.);
#1353=FACE_BOUND('',#4090,.T.);
#1354=FACE_BOUND('',#4091,.T.);
#1355=FACE_BOUND('',#4092,.T.);
#1356=FACE_BOUND('',#4093,.T.);
#1357=FACE_BOUND('',#4094,.T.);
#1358=FACE_BOUND('',#4095,.T.);
#1359=FACE_BOUND('',#4096,.T.);
#1360=FACE_BOUND('',#4097,.T.);
#1361=FACE_BOUND('',#4098,.T.);
#1362=FACE_BOUND('',#4099,.T.);
#1363=FACE_BOUND('',#4100,.T.);
#1364=FACE_BOUND('',#4101,.T.);
#1365=FACE_BOUND('',#4102,.T.);
#1366=FACE_BOUND('',#4103,.T.);
#1367=FACE_BOUND('',#4104,.T.);
#1368=FACE_BOUND('',#4105,.T.);
#1369=FACE_BOUND('',#4107,.T.);
#1370=FACE_BOUND('',#4111,.T.);
#1371=FACE_BOUND('',#4119,.T.);
#1372=FACE_BOUND('',#4121,.T.);
#1373=FACE_BOUND('',#4122,.T.);
#1374=FACE_BOUND('',#4123,.T.);
#1375=FACE_BOUND('',#4124,.T.);
#1376=FACE_BOUND('',#4125,.T.);
#1377=FACE_BOUND('',#4131,.T.);
#1378=FACE_BOUND('',#4132,.T.);
#1379=FACE_BOUND('',#4133,.T.);
#1380=FACE_BOUND('',#4134,.T.);
#1381=FACE_BOUND('',#4135,.T.);
#1553=PLANE('',#24132);
#1554=PLANE('',#24147);
#1555=PLANE('',#24148);
#1556=PLANE('',#24150);
#1557=PLANE('',#24151);
#1558=PLANE('',#24153);
#1559=PLANE('',#24154);
#1560=PLANE('',#24156);
#1561=PLANE('',#24157);
#1562=PLANE('',#24159);
#1563=PLANE('',#24160);
#1564=PLANE('',#24162);
#1565=PLANE('',#24163);
#1566=PLANE('',#24165);
#1567=PLANE('',#24166);
#1568=PLANE('',#24168);
#1569=PLANE('',#24169);
#1570=PLANE('',#24171);
#1571=PLANE('',#24172);
#1572=PLANE('',#24174);
#1573=PLANE('',#24175);
#1574=PLANE('',#24177);
#1575=PLANE('',#24178);
#1576=PLANE('',#24180);
#1577=PLANE('',#24181);
#1578=PLANE('',#24183);
#1579=PLANE('',#24184);
#1580=PLANE('',#24186);
#1581=PLANE('',#24187);
#1582=PLANE('',#24189);
#1583=PLANE('',#24190);
#1584=PLANE('',#24192);
#1585=PLANE('',#24193);
#1586=PLANE('',#24195);
#1587=PLANE('',#24196);
#1588=PLANE('',#24198);
#1589=PLANE('',#24199);
#1590=PLANE('',#24201);
#1591=PLANE('',#24202);
#1592=PLANE('',#24204);
#1593=PLANE('',#24205);
#1594=PLANE('',#24207);
#1595=PLANE('',#24208);
#1596=PLANE('',#24210);
#1597=PLANE('',#24211);
#1598=PLANE('',#24213);
#1599=PLANE('',#24214);
#1600=PLANE('',#24217);
#1601=PLANE('',#24218);
#1602=PLANE('',#24221);
#1603=PLANE('',#24222);
#1604=PLANE('',#24224);
#1605=PLANE('',#24225);
#1606=PLANE('',#24227);
#1607=PLANE('',#24228);
#1608=PLANE('',#24230);
#1609=PLANE('',#24231);
#1610=PLANE('',#24233);
#1611=PLANE('',#24234);
#1612=PLANE('',#24236);
#1613=PLANE('',#24237);
#1614=PLANE('',#24239);
#1615=PLANE('',#24240);
#1616=PLANE('',#24242);
#1617=PLANE('',#24243);
#1618=PLANE('',#24245);
#1619=PLANE('',#24246);
#1620=PLANE('',#24248);
#1621=PLANE('',#24249);
#1622=PLANE('',#24251);
#1623=PLANE('',#24252);
#1624=PLANE('',#24254);
#1625=PLANE('',#24255);
#1626=PLANE('',#24257);
#1627=PLANE('',#24258);
#1628=PLANE('',#24260);
#1629=PLANE('',#24261);
#1630=PLANE('',#24263);
#1631=PLANE('',#24264);
#1632=PLANE('',#24266);
#1633=PLANE('',#24267);
#1634=PLANE('',#24269);
#1635=PLANE('',#24270);
#1636=PLANE('',#24272);
#1637=PLANE('',#24273);
#1638=PLANE('',#24275);
#1639=PLANE('',#24276);
#1640=PLANE('',#24278);
#1641=PLANE('',#24279);
#1642=PLANE('',#24281);
#1643=PLANE('',#24282);
#1644=PLANE('',#24284);
#1645=PLANE('',#24285);
#1646=PLANE('',#24287);
#1647=PLANE('',#24288);
#1648=PLANE('',#24290);
#1649=PLANE('',#24291);
#1650=PLANE('',#24298);
#1651=PLANE('',#24299);
#1652=PLANE('',#24306);
#1653=PLANE('',#24312);
#1654=PLANE('',#24313);
#1655=PLANE('',#24314);
#1656=PLANE('',#24315);
#1657=PLANE('',#24316);
#1658=PLANE('',#24317);
#1659=PLANE('',#24318);
#1660=PLANE('',#24319);
#1661=PLANE('',#24320);
#1662=PLANE('',#24322);
#1663=PLANE('',#24323);
#1664=PLANE('',#24324);
#1665=PLANE('',#24325);
#1666=PLANE('',#24326);
#1667=PLANE('',#24327);
#2555=FACE_OUTER_BOUND('',#3951,.T.);
#2556=FACE_OUTER_BOUND('',#3952,.T.);
#2557=FACE_OUTER_BOUND('',#3953,.T.);
#2558=FACE_OUTER_BOUND('',#3954,.T.);
#2559=FACE_OUTER_BOUND('',#3955,.T.);
#2560=FACE_OUTER_BOUND('',#3956,.T.);
#2561=FACE_OUTER_BOUND('',#3957,.T.);
#2562=FACE_OUTER_BOUND('',#3958,.T.);
#2563=FACE_OUTER_BOUND('',#3959,.T.);
#2564=FACE_OUTER_BOUND('',#3960,.T.);
#2565=FACE_OUTER_BOUND('',#3961,.T.);
#2566=FACE_OUTER_BOUND('',#3962,.T.);
#2567=FACE_OUTER_BOUND('',#3963,.T.);
#2568=FACE_OUTER_BOUND('',#3964,.T.);
#2569=FACE_OUTER_BOUND('',#3965,.T.);
#2570=FACE_OUTER_BOUND('',#3966,.T.);
#2571=FACE_OUTER_BOUND('',#3967,.T.);
#2572=FACE_OUTER_BOUND('',#3968,.T.);
#2573=FACE_OUTER_BOUND('',#3969,.T.);
#2574=FACE_OUTER_BOUND('',#3970,.T.);
#2575=FACE_OUTER_BOUND('',#3971,.T.);
#2576=FACE_OUTER_BOUND('',#3972,.T.);
#2577=FACE_OUTER_BOUND('',#3973,.T.);
#2578=FACE_OUTER_BOUND('',#3974,.T.);
#2579=FACE_OUTER_BOUND('',#3975,.T.);
#2580=FACE_OUTER_BOUND('',#3976,.T.);
#2581=FACE_OUTER_BOUND('',#3977,.T.);
#2582=FACE_OUTER_BOUND('',#3978,.T.);
#2583=FACE_OUTER_BOUND('',#3979,.T.);
#2584=FACE_OUTER_BOUND('',#3980,.T.);
#2585=FACE_OUTER_BOUND('',#3981,.T.);
#2586=FACE_OUTER_BOUND('',#3982,.T.);
#2587=FACE_OUTER_BOUND('',#3983,.T.);
#2588=FACE_OUTER_BOUND('',#3984,.T.);
#2589=FACE_OUTER_BOUND('',#3985,.T.);
#2590=FACE_OUTER_BOUND('',#3986,.T.);
#2591=FACE_OUTER_BOUND('',#3987,.T.);
#2592=FACE_OUTER_BOUND('',#3988,.T.);
#2593=FACE_OUTER_BOUND('',#3989,.T.);
#2594=FACE_OUTER_BOUND('',#3990,.T.);
#2595=FACE_OUTER_BOUND('',#3991,.T.);
#2596=FACE_OUTER_BOUND('',#3992,.T.);
#2597=FACE_OUTER_BOUND('',#3993,.T.);
#2598=FACE_OUTER_BOUND('',#3994,.T.);
#2599=FACE_OUTER_BOUND('',#3995,.T.);
#2600=FACE_OUTER_BOUND('',#3996,.T.);
#2601=FACE_OUTER_BOUND('',#3997,.T.);
#2602=FACE_OUTER_BOUND('',#3998,.T.);
#2603=FACE_OUTER_BOUND('',#3999,.T.);
#2604=FACE_OUTER_BOUND('',#4000,.T.);
#2605=FACE_OUTER_BOUND('',#4001,.T.);
#2606=FACE_OUTER_BOUND('',#4002,.T.);
#2607=FACE_OUTER_BOUND('',#4003,.T.);
#2608=FACE_OUTER_BOUND('',#4004,.T.);
#2609=FACE_OUTER_BOUND('',#4005,.T.);
#2610=FACE_OUTER_BOUND('',#4006,.T.);
#2611=FACE_OUTER_BOUND('',#4007,.T.);
#2612=FACE_OUTER_BOUND('',#4008,.T.);
#2613=FACE_OUTER_BOUND('',#4009,.T.);
#2614=FACE_OUTER_BOUND('',#4010,.T.);
#2615=FACE_OUTER_BOUND('',#4011,.T.);
#2616=FACE_OUTER_BOUND('',#4012,.T.);
#2617=FACE_OUTER_BOUND('',#4013,.T.);
#2618=FACE_OUTER_BOUND('',#4014,.T.);
#2619=FACE_OUTER_BOUND('',#4015,.T.);
#2620=FACE_OUTER_BOUND('',#4016,.T.);
#2621=FACE_OUTER_BOUND('',#4017,.T.);
#2622=FACE_OUTER_BOUND('',#4018,.T.);
#2623=FACE_OUTER_BOUND('',#4019,.T.);
#2624=FACE_OUTER_BOUND('',#4020,.T.);
#2625=FACE_OUTER_BOUND('',#4021,.T.);
#2626=FACE_OUTER_BOUND('',#4022,.T.);
#2627=FACE_OUTER_BOUND('',#4023,.T.);
#2628=FACE_OUTER_BOUND('',#4024,.T.);
#2629=FACE_OUTER_BOUND('',#4025,.T.);
#2630=FACE_OUTER_BOUND('',#4026,.T.);
#2631=FACE_OUTER_BOUND('',#4027,.T.);
#2632=FACE_OUTER_BOUND('',#4028,.T.);
#2633=FACE_OUTER_BOUND('',#4029,.T.);
#2634=FACE_OUTER_BOUND('',#4030,.T.);
#2635=FACE_OUTER_BOUND('',#4031,.T.);
#2636=FACE_OUTER_BOUND('',#4032,.T.);
#2637=FACE_OUTER_BOUND('',#4033,.T.);
#2638=FACE_OUTER_BOUND('',#4034,.T.);
#2639=FACE_OUTER_BOUND('',#4035,.T.);
#2640=FACE_OUTER_BOUND('',#4036,.T.);
#2641=FACE_OUTER_BOUND('',#4037,.T.);
#2642=FACE_OUTER_BOUND('',#4038,.T.);
#2643=FACE_OUTER_BOUND('',#4039,.T.);
#2644=FACE_OUTER_BOUND('',#4040,.T.);
#2645=FACE_OUTER_BOUND('',#4041,.T.);
#2646=FACE_OUTER_BOUND('',#4042,.T.);
#2647=FACE_OUTER_BOUND('',#4043,.T.);
#2648=FACE_OUTER_BOUND('',#4044,.T.);
#2649=FACE_OUTER_BOUND('',#4045,.T.);
#2650=FACE_OUTER_BOUND('',#4046,.T.);
#2651=FACE_OUTER_BOUND('',#4047,.T.);
#2652=FACE_OUTER_BOUND('',#4048,.T.);
#2653=FACE_OUTER_BOUND('',#4049,.T.);
#2654=FACE_OUTER_BOUND('',#4050,.T.);
#2655=FACE_OUTER_BOUND('',#4051,.T.);
#2656=FACE_OUTER_BOUND('',#4052,.T.);
#2657=FACE_OUTER_BOUND('',#4053,.T.);
#2658=FACE_OUTER_BOUND('',#4054,.T.);
#2659=FACE_OUTER_BOUND('',#4055,.T.);
#2660=FACE_OUTER_BOUND('',#4056,.T.);
#2661=FACE_OUTER_BOUND('',#4057,.T.);
#2662=FACE_OUTER_BOUND('',#4058,.T.);
#2663=FACE_OUTER_BOUND('',#4059,.T.);
#2664=FACE_OUTER_BOUND('',#4060,.T.);
#2665=FACE_OUTER_BOUND('',#4061,.T.);
#2666=FACE_OUTER_BOUND('',#4062,.T.);
#2667=FACE_OUTER_BOUND('',#4063,.T.);
#2668=FACE_OUTER_BOUND('',#4064,.T.);
#2669=FACE_OUTER_BOUND('',#4065,.T.);
#2670=FACE_OUTER_BOUND('',#4066,.T.);
#2671=FACE_OUTER_BOUND('',#4067,.T.);
#2672=FACE_OUTER_BOUND('',#4068,.T.);
#2673=FACE_OUTER_BOUND('',#4069,.T.);
#2674=FACE_OUTER_BOUND('',#4070,.T.);
#2675=FACE_OUTER_BOUND('',#4071,.T.);
#2676=FACE_OUTER_BOUND('',#4072,.T.);
#2677=FACE_OUTER_BOUND('',#4073,.T.);
#2678=FACE_OUTER_BOUND('',#4074,.T.);
#2679=FACE_OUTER_BOUND('',#4075,.T.);
#2680=FACE_OUTER_BOUND('',#4076,.T.);
#2681=FACE_OUTER_BOUND('',#4077,.T.);
#2682=FACE_OUTER_BOUND('',#4078,.T.);
#2683=FACE_OUTER_BOUND('',#4079,.T.);
#2684=FACE_OUTER_BOUND('',#4081,.T.);
#2685=FACE_OUTER_BOUND('',#4082,.T.);
#2686=FACE_OUTER_BOUND('',#4106,.T.);
#2687=FACE_OUTER_BOUND('',#4108,.T.);
#2688=FACE_OUTER_BOUND('',#4109,.T.);
#2689=FACE_OUTER_BOUND('',#4110,.T.);
#2690=FACE_OUTER_BOUND('',#4112,.T.);
#2691=FACE_OUTER_BOUND('',#4113,.T.);
#2692=FACE_OUTER_BOUND('',#4114,.T.);
#2693=FACE_OUTER_BOUND('',#4115,.T.);
#2694=FACE_OUTER_BOUND('',#4116,.T.);
#2695=FACE_OUTER_BOUND('',#4117,.T.);
#2696=FACE_OUTER_BOUND('',#4118,.T.);
#2697=FACE_OUTER_BOUND('',#4120,.T.);
#2698=FACE_OUTER_BOUND('',#4126,.T.);
#2699=FACE_OUTER_BOUND('',#4127,.T.);
#2700=FACE_OUTER_BOUND('',#4128,.T.);
#2701=FACE_OUTER_BOUND('',#4129,.T.);
#2702=FACE_OUTER_BOUND('',#4130,.T.);
#2703=FACE_OUTER_BOUND('',#4136,.T.);
#2704=FACE_OUTER_BOUND('',#4137,.T.);
#2705=FACE_OUTER_BOUND('',#4138,.T.);
#3951=EDGE_LOOP('',(#16447,#16448,#16449,#16450,#16451,#16452,#16453,#16454));
#3952=EDGE_LOOP('',(#16455,#16456,#16457,#16458));
#3953=EDGE_LOOP('',(#16459,#16460,#16461,#16462));
#3954=EDGE_LOOP('',(#16463,#16464,#16465,#16466));
#3955=EDGE_LOOP('',(#16467,#16468,#16469,#16470));
#3956=EDGE_LOOP('',(#16471,#16472,#16473,#16474));
#3957=EDGE_LOOP('',(#16475,#16476,#16477,#16478));
#3958=EDGE_LOOP('',(#16479,#16480,#16481,#16482));
#3959=EDGE_LOOP('',(#16483,#16484,#16485,#16486));
#3960=EDGE_LOOP('',(#16487,#16488,#16489,#16490));
#3961=EDGE_LOOP('',(#16491,#16492,#16493,#16494));
#3962=EDGE_LOOP('',(#16495,#16496,#16497,#16498));
#3963=EDGE_LOOP('',(#16499,#16500,#16501,#16502));
#3964=EDGE_LOOP('',(#16503,#16504,#16505,#16506));
#3965=EDGE_LOOP('',(#16507,#16508,#16509,#16510));
#3966=EDGE_LOOP('',(#16511,#16512,#16513,#16514));
#3967=EDGE_LOOP('',(#16515,#16516,#16517,#16518));
#3968=EDGE_LOOP('',(#16519,#16520,#16521,#16522));
#3969=EDGE_LOOP('',(#16523,#16524,#16525,#16526));
#3970=EDGE_LOOP('',(#16527,#16528,#16529,#16530));
#3971=EDGE_LOOP('',(#16531,#16532,#16533,#16534));
#3972=EDGE_LOOP('',(#16535,#16536,#16537,#16538,#16539,#16540,#16541,#16542,
#16543,#16544,#16545,#16546,#16547,#16548,#16549,#16550,#16551,#16552,#16553,
#16554,#16555,#16556,#16557,#16558,#16559));
#3973=EDGE_LOOP('',(#16560,#16561,#16562,#16563));
#3974=EDGE_LOOP('',(#16564,#16565,#16566,#16567));
#3975=EDGE_LOOP('',(#16568,#16569,#16570,#16571,#16572,#16573,#16574,#16575,
#16576,#16577,#16578,#16579,#16580,#16581,#16582,#16583,#16584,#16585,#16586,
#16587,#16588,#16589,#16590,#16591,#16592,#16593));
#3976=EDGE_LOOP('',(#16594,#16595,#16596,#16597));
#3977=EDGE_LOOP('',(#16598,#16599,#16600,#16601));
#3978=EDGE_LOOP('',(#16602,#16603,#16604,#16605));
#3979=EDGE_LOOP('',(#16606,#16607,#16608,#16609));
#3980=EDGE_LOOP('',(#16610,#16611,#16612,#16613));
#3981=EDGE_LOOP('',(#16614,#16615,#16616));
#3982=EDGE_LOOP('',(#16617,#16618,#16619,#16620));
#3983=EDGE_LOOP('',(#16621,#16622,#16623));
#3984=EDGE_LOOP('',(#16624,#16625,#16626,#16627));
#3985=EDGE_LOOP('',(#16628,#16629,#16630));
#3986=EDGE_LOOP('',(#16631,#16632,#16633,#16634));
#3987=EDGE_LOOP('',(#16635,#16636,#16637));
#3988=EDGE_LOOP('',(#16638,#16639,#16640,#16641));
#3989=EDGE_LOOP('',(#16642,#16643,#16644));
#3990=EDGE_LOOP('',(#16645,#16646,#16647,#16648));
#3991=EDGE_LOOP('',(#16649,#16650,#16651));
#3992=EDGE_LOOP('',(#16652,#16653,#16654,#16655));
#3993=EDGE_LOOP('',(#16656,#16657,#16658));
#3994=EDGE_LOOP('',(#16659,#16660,#16661,#16662));
#3995=EDGE_LOOP('',(#16663,#16664,#16665));
#3996=EDGE_LOOP('',(#16666,#16667,#16668,#16669));
#3997=EDGE_LOOP('',(#16670,#16671,#16672));
#3998=EDGE_LOOP('',(#16673,#16674,#16675,#16676));
#3999=EDGE_LOOP('',(#16677,#16678,#16679));
#4000=EDGE_LOOP('',(#16680,#16681,#16682,#16683));
#4001=EDGE_LOOP('',(#16684,#16685,#16686));
#4002=EDGE_LOOP('',(#16687,#16688,#16689,#16690));
#4003=EDGE_LOOP('',(#16691,#16692,#16693));
#4004=EDGE_LOOP('',(#16694,#16695,#16696,#16697));
#4005=EDGE_LOOP('',(#16698,#16699,#16700));
#4006=EDGE_LOOP('',(#16701,#16702,#16703,#16704));
#4007=EDGE_LOOP('',(#16705,#16706,#16707));
#4008=EDGE_LOOP('',(#16708,#16709,#16710,#16711));
#4009=EDGE_LOOP('',(#16712,#16713,#16714));
#4010=EDGE_LOOP('',(#16715,#16716,#16717,#16718));
#4011=EDGE_LOOP('',(#16719,#16720,#16721));
#4012=EDGE_LOOP('',(#16722,#16723,#16724,#16725));
#4013=EDGE_LOOP('',(#16726,#16727,#16728));
#4014=EDGE_LOOP('',(#16729,#16730,#16731,#16732));
#4015=EDGE_LOOP('',(#16733,#16734,#16735));
#4016=EDGE_LOOP('',(#16736,#16737,#16738,#16739));
#4017=EDGE_LOOP('',(#16740,#16741,#16742));
#4018=EDGE_LOOP('',(#16743,#16744,#16745,#16746));
#4019=EDGE_LOOP('',(#16747,#16748,#16749));
#4020=EDGE_LOOP('',(#16750,#16751,#16752,#16753));
#4021=EDGE_LOOP('',(#16754,#16755,#16756));
#4022=EDGE_LOOP('',(#16757,#16758,#16759,#16760));
#4023=EDGE_LOOP('',(#16761,#16762,#16763));
#4024=EDGE_LOOP('',(#16764,#16765,#16766,#16767));
#4025=EDGE_LOOP('',(#16768,#16769,#16770,#16771));
#4026=EDGE_LOOP('',(#16772,#16773,#16774,#16775));
#4027=EDGE_LOOP('',(#16776,#16777,#16778,#16779));
#4028=EDGE_LOOP('',(#16780,#16781,#16782,#16783));
#4029=EDGE_LOOP('',(#16784,#16785,#16786));
#4030=EDGE_LOOP('',(#16787,#16788,#16789,#16790));
#4031=EDGE_LOOP('',(#16791,#16792,#16793));
#4032=EDGE_LOOP('',(#16794,#16795,#16796,#16797));
#4033=EDGE_LOOP('',(#16798,#16799,#16800));
#4034=EDGE_LOOP('',(#16801,#16802,#16803,#16804));
#4035=EDGE_LOOP('',(#16805,#16806,#16807));
#4036=EDGE_LOOP('',(#16808,#16809,#16810,#16811));
#4037=EDGE_LOOP('',(#16812,#16813,#16814));
#4038=EDGE_LOOP('',(#16815,#16816,#16817,#16818));
#4039=EDGE_LOOP('',(#16819,#16820,#16821));
#4040=EDGE_LOOP('',(#16822,#16823,#16824,#16825));
#4041=EDGE_LOOP('',(#16826,#16827,#16828));
#4042=EDGE_LOOP('',(#16829,#16830,#16831,#16832));
#4043=EDGE_LOOP('',(#16833,#16834,#16835));
#4044=EDGE_LOOP('',(#16836,#16837,#16838,#16839));
#4045=EDGE_LOOP('',(#16840,#16841,#16842));
#4046=EDGE_LOOP('',(#16843,#16844,#16845,#16846));
#4047=EDGE_LOOP('',(#16847,#16848,#16849));
#4048=EDGE_LOOP('',(#16850,#16851,#16852,#16853));
#4049=EDGE_LOOP('',(#16854,#16855,#16856));
#4050=EDGE_LOOP('',(#16857,#16858,#16859,#16860));
#4051=EDGE_LOOP('',(#16861,#16862,#16863));
#4052=EDGE_LOOP('',(#16864,#16865,#16866,#16867));
#4053=EDGE_LOOP('',(#16868,#16869,#16870));
#4054=EDGE_LOOP('',(#16871,#16872,#16873,#16874));
#4055=EDGE_LOOP('',(#16875,#16876,#16877));
#4056=EDGE_LOOP('',(#16878,#16879,#16880,#16881));
#4057=EDGE_LOOP('',(#16882,#16883,#16884));
#4058=EDGE_LOOP('',(#16885,#16886,#16887,#16888));
#4059=EDGE_LOOP('',(#16889,#16890,#16891));
#4060=EDGE_LOOP('',(#16892,#16893,#16894,#16895));
#4061=EDGE_LOOP('',(#16896,#16897,#16898));
#4062=EDGE_LOOP('',(#16899,#16900,#16901,#16902));
#4063=EDGE_LOOP('',(#16903,#16904,#16905));
#4064=EDGE_LOOP('',(#16906,#16907,#16908,#16909));
#4065=EDGE_LOOP('',(#16910,#16911,#16912));
#4066=EDGE_LOOP('',(#16913,#16914,#16915,#16916));
#4067=EDGE_LOOP('',(#16917,#16918,#16919));
#4068=EDGE_LOOP('',(#16920,#16921,#16922,#16923));
#4069=EDGE_LOOP('',(#16924,#16925,#16926));
#4070=EDGE_LOOP('',(#16927,#16928,#16929,#16930));
#4071=EDGE_LOOP('',(#16931,#16932,#16933));
#4072=EDGE_LOOP('',(#16934,#16935,#16936,#16937));
#4073=EDGE_LOOP('',(#16938,#16939,#16940));
#4074=EDGE_LOOP('',(#16941,#16942,#16943,#16944));
#4075=EDGE_LOOP('',(#16945,#16946,#16947));
#4076=EDGE_LOOP('',(#16948,#16949,#16950,#16951));
#4077=EDGE_LOOP('',(#16952,#16953,#16954,#16955));
#4078=EDGE_LOOP('',(#16956));
#4079=EDGE_LOOP('',(#16957));
#4080=EDGE_LOOP('',(#16958));
#4081=EDGE_LOOP('',(#16959,#16960,#16961,#16962));
#4082=EDGE_LOOP('',(#16963,#16964,#16965,#16966,#16967,#16968,#16969,#16970,
#16971,#16972,#16973,#16974));
#4083=EDGE_LOOP('',(#16975,#16976,#16977,#16978));
#4084=EDGE_LOOP('',(#16979,#16980,#16981,#16982));
#4085=EDGE_LOOP('',(#16983,#16984,#16985,#16986));
#4086=EDGE_LOOP('',(#16987,#16988,#16989,#16990));
#4087=EDGE_LOOP('',(#16991,#16992,#16993,#16994));
#4088=EDGE_LOOP('',(#16995,#16996,#16997,#16998));
#4089=EDGE_LOOP('',(#16999,#17000,#17001,#17002));
#4090=EDGE_LOOP('',(#17003,#17004,#17005,#17006));
#4091=EDGE_LOOP('',(#17007,#17008,#17009,#17010));
#4092=EDGE_LOOP('',(#17011,#17012,#17013,#17014));
#4093=EDGE_LOOP('',(#17015,#17016,#17017,#17018));
#4094=EDGE_LOOP('',(#17019,#17020,#17021,#17022));
#4095=EDGE_LOOP('',(#17023,#17024,#17025,#17026));
#4096=EDGE_LOOP('',(#17027,#17028,#17029,#17030));
#4097=EDGE_LOOP('',(#17031,#17032,#17033,#17034));
#4098=EDGE_LOOP('',(#17035,#17036,#17037,#17038));
#4099=EDGE_LOOP('',(#17039,#17040,#17041,#17042));
#4100=EDGE_LOOP('',(#17043,#17044,#17045,#17046));
#4101=EDGE_LOOP('',(#17047,#17048,#17049,#17050));
#4102=EDGE_LOOP('',(#17051,#17052,#17053,#17054));
#4103=EDGE_LOOP('',(#17055,#17056,#17057,#17058));
#4104=EDGE_LOOP('',(#17059,#17060,#17061,#17062));
#4105=EDGE_LOOP('',(#17063,#17064,#17065,#17066));
#4106=EDGE_LOOP('',(#17067));
#4107=EDGE_LOOP('',(#17068));
#4108=EDGE_LOOP('',(#17069,#17070,#17071,#17072));
#4109=EDGE_LOOP('',(#17073,#17074,#17075,#17076));
#4110=EDGE_LOOP('',(#17077));
#4111=EDGE_LOOP('',(#17078));
#4112=EDGE_LOOP('',(#17079,#17080,#17081,#17082));
#4113=EDGE_LOOP('',(#17083,#17084,#17085,#17086));
#4114=EDGE_LOOP('',(#17087,#17088,#17089,#17090));
#4115=EDGE_LOOP('',(#17091,#17092,#17093,#17094));
#4116=EDGE_LOOP('',(#17095,#17096,#17097,#17098));
#4117=EDGE_LOOP('',(#17099,#17100,#17101,#17102));
#4118=EDGE_LOOP('',(#17103,#17104,#17105,#17106,#17107,#17108));
#4119=EDGE_LOOP('',(#17109));
#4120=EDGE_LOOP('',(#17110,#17111,#17112,#17113));
#4121=EDGE_LOOP('',(#17114));
#4122=EDGE_LOOP('',(#17115));
#4123=EDGE_LOOP('',(#17116));
#4124=EDGE_LOOP('',(#17117));
#4125=EDGE_LOOP('',(#17118,#17119,#17120,#17121));
#4126=EDGE_LOOP('',(#17122,#17123,#17124,#17125));
#4127=EDGE_LOOP('',(#17126,#17127,#17128,#17129));
#4128=EDGE_LOOP('',(#17130,#17131,#17132,#17133));
#4129=EDGE_LOOP('',(#17134,#17135,#17136,#17137));
#4130=EDGE_LOOP('',(#17138,#17139,#17140,#17141));
#4131=EDGE_LOOP('',(#17142));
#4132=EDGE_LOOP('',(#17143));
#4133=EDGE_LOOP('',(#17144));
#4134=EDGE_LOOP('',(#17145));
#4135=EDGE_LOOP('',(#17146,#17147,#17148,#17149,#17150,#17151));
#4136=EDGE_LOOP('',(#17152));
#4137=EDGE_LOOP('',(#17153,#17154,#17155,#17156));
#4138=EDGE_LOOP('',(#17157,#17158,#17159,#17160));
#5349=CIRCLE('',#24109,0.3954);
#5350=CIRCLE('',#24110,0.3954);
#5351=CIRCLE('',#24121,0.352375);
#5352=CIRCLE('',#24133,0.352375);
#5353=CIRCLE('',#24136,0.08);
#5354=CIRCLE('',#24137,0.08);
#5355=CIRCLE('',#24139,0.08);
#5356=CIRCLE('',#24140,0.08);
#5357=CIRCLE('',#24142,0.08);
#5358=CIRCLE('',#24143,0.08);
#5359=CIRCLE('',#24145,0.08);
#5360=CIRCLE('',#24146,0.08);
#5361=CIRCLE('',#24149,0.5);
#5362=CIRCLE('',#24152,0.5);
#5363=CIRCLE('',#24155,0.5);
#5364=CIRCLE('',#24158,0.5);
#5365=CIRCLE('',#24161,0.5);
#5366=CIRCLE('',#24164,0.5);
#5367=CIRCLE('',#24167,0.5);
#5368=CIRCLE('',#24170,0.5);
#5369=CIRCLE('',#24173,0.5);
#5370=CIRCLE('',#24176,0.5);
#5371=CIRCLE('',#24179,0.5);
#5372=CIRCLE('',#24182,0.5);
#5373=CIRCLE('',#24185,0.5);
#5374=CIRCLE('',#24188,0.5);
#5375=CIRCLE('',#24191,0.5);
#5376=CIRCLE('',#24194,0.5);
#5377=CIRCLE('',#24197,0.5);
#5378=CIRCLE('',#24200,0.5);
#5379=CIRCLE('',#24203,0.5);
#5380=CIRCLE('',#24206,0.5);
#5381=CIRCLE('',#24209,0.5);
#5382=CIRCLE('',#24212,0.5);
#5383=CIRCLE('',#24215,0.5);
#5384=CIRCLE('',#24216,0.5);
#5385=CIRCLE('',#24219,0.5);
#5386=CIRCLE('',#24220,0.5);
#5387=CIRCLE('',#24223,0.5);
#5388=CIRCLE('',#24226,0.5);
#5389=CIRCLE('',#24229,0.5);
#5390=CIRCLE('',#24232,0.5);
#5391=CIRCLE('',#24235,0.5);
#5392=CIRCLE('',#24238,0.5);
#5393=CIRCLE('',#24241,0.5);
#5394=CIRCLE('',#24244,0.5);
#5395=CIRCLE('',#24247,0.5);
#5396=CIRCLE('',#24250,0.5);
#5397=CIRCLE('',#24253,0.5);
#5398=CIRCLE('',#24256,0.5);
#5399=CIRCLE('',#24259,0.5);
#5400=CIRCLE('',#24262,0.5);
#5401=CIRCLE('',#24265,0.5);
#5402=CIRCLE('',#24268,0.5);
#5403=CIRCLE('',#24271,0.5);
#5404=CIRCLE('',#24274,0.5);
#5405=CIRCLE('',#24277,0.5);
#5406=CIRCLE('',#24280,0.5);
#5407=CIRCLE('',#24283,0.5);
#5408=CIRCLE('',#24286,0.5);
#5409=CIRCLE('',#24289,0.5);
#5410=CIRCLE('',#24292,0.5);
#5411=CIRCLE('',#24294,0.06);
#5412=CIRCLE('',#24295,0.06);
#5413=CIRCLE('',#24297,0.03);
#5414=CIRCLE('',#24300,0.25);
#5415=CIRCLE('',#24302,0.25);
#5416=CIRCLE('',#24304,0.5);
#5417=CIRCLE('',#24305,0.5);
#5418=CIRCLE('',#24307,0.52);
#5419=CIRCLE('',#24309,0.52);
#5420=CIRCLE('',#24311,0.48);
#5421=CIRCLE('',#24321,0.3954);
#5422=CIRCLE('',#24328,0.36);
#6256=LINE('',#33237,#8101);
#6257=LINE('',#33265,#8102);
#6258=LINE('',#33299,#8103);
#6259=LINE('',#33347,#8104);
#6260=LINE('',#33395,#8105);
#6261=LINE('',#33443,#8106);
#6262=LINE('',#33491,#8107);
#6263=LINE('',#33545,#8108);
#6264=LINE('',#33593,#8109);
#6265=LINE('',#33641,#8110);
#6266=LINE('',#33695,#8111);
#6267=LINE('',#33743,#8112);
#6268=LINE('',#33759,#8113);
#6269=LINE('',#33783,#8114);
#6270=LINE('',#33808,#8115);
#6271=LINE('',#33833,#8116);
#6272=LINE('',#33857,#8117);
#6273=LINE('',#33882,#8118);
#6274=LINE('',#33907,#8119);
#6275=LINE('',#33931,#8120);
#6276=LINE('',#33957,#8121);
#6277=LINE('',#33981,#8122);
#6278=LINE('',#34891,#8123);
#6279=LINE('',#34897,#8124);
#6280=LINE('',#34903,#8125);
#6281=LINE('',#34909,#8126);
#6282=LINE('',#34914,#8127);
#6283=LINE('',#34916,#8128);
#6284=LINE('',#34918,#8129);
#6285=LINE('',#34919,#8130);
#6286=LINE('',#34923,#8131);
#6287=LINE('',#34926,#8132);
#6288=LINE('',#34927,#8133);
#6289=LINE('',#34933,#8134);
#6290=LINE('',#34935,#8135);
#6291=LINE('',#34937,#8136);
#6292=LINE('',#34938,#8137);
#6293=LINE('',#34942,#8138);
#6294=LINE('',#34945,#8139);
#6295=LINE('',#34946,#8140);
#6296=LINE('',#34952,#8141);
#6297=LINE('',#34954,#8142);
#6298=LINE('',#34956,#8143);
#6299=LINE('',#34957,#8144);
#6300=LINE('',#34961,#8145);
#6301=LINE('',#34964,#8146);
#6302=LINE('',#34965,#8147);
#6303=LINE('',#34971,#8148);
#6304=LINE('',#34973,#8149);
#6305=LINE('',#34975,#8150);
#6306=LINE('',#34976,#8151);
#6307=LINE('',#34980,#8152);
#6308=LINE('',#34983,#8153);
#6309=LINE('',#34984,#8154);
#6310=LINE('',#34990,#8155);
#6311=LINE('',#34992,#8156);
#6312=LINE('',#34994,#8157);
#6313=LINE('',#34995,#8158);
#6314=LINE('',#34999,#8159);
#6315=LINE('',#35002,#8160);
#6316=LINE('',#35003,#8161);
#6317=LINE('',#35009,#8162);
#6318=LINE('',#35011,#8163);
#6319=LINE('',#35013,#8164);
#6320=LINE('',#35014,#8165);
#6321=LINE('',#35018,#8166);
#6322=LINE('',#35021,#8167);
#6323=LINE('',#35022,#8168);
#6324=LINE('',#35028,#8169);
#6325=LINE('',#35030,#8170);
#6326=LINE('',#35032,#8171);
#6327=LINE('',#35033,#8172);
#6328=LINE('',#35037,#8173);
#6329=LINE('',#35040,#8174);
#6330=LINE('',#35041,#8175);
#6331=LINE('',#35047,#8176);
#6332=LINE('',#35049,#8177);
#6333=LINE('',#35051,#8178);
#6334=LINE('',#35052,#8179);
#6335=LINE('',#35056,#8180);
#6336=LINE('',#35059,#8181);
#6337=LINE('',#35060,#8182);
#6338=LINE('',#35066,#8183);
#6339=LINE('',#35068,#8184);
#6340=LINE('',#35070,#8185);
#6341=LINE('',#35071,#8186);
#6342=LINE('',#35075,#8187);
#6343=LINE('',#35078,#8188);
#6344=LINE('',#35079,#8189);
#6345=LINE('',#35085,#8190);
#6346=LINE('',#35087,#8191);
#6347=LINE('',#35089,#8192);
#6348=LINE('',#35090,#8193);
#6349=LINE('',#35094,#8194);
#6350=LINE('',#35097,#8195);
#6351=LINE('',#35098,#8196);
#6352=LINE('',#35104,#8197);
#6353=LINE('',#35106,#8198);
#6354=LINE('',#35108,#8199);
#6355=LINE('',#35109,#8200);
#6356=LINE('',#35113,#8201);
#6357=LINE('',#35116,#8202);
#6358=LINE('',#35117,#8203);
#6359=LINE('',#35123,#8204);
#6360=LINE('',#35125,#8205);
#6361=LINE('',#35127,#8206);
#6362=LINE('',#35128,#8207);
#6363=LINE('',#35133,#8208);
#6364=LINE('',#35137,#8209);
#6365=LINE('',#35138,#8210);
#6366=LINE('',#35146,#8211);
#6367=LINE('',#35148,#8212);
#6368=LINE('',#35150,#8213);
#6369=LINE('',#35151,#8214);
#6370=LINE('',#35155,#8215);
#6371=LINE('',#35158,#8216);
#6372=LINE('',#35159,#8217);
#6373=LINE('',#35165,#8218);
#6374=LINE('',#35167,#8219);
#6375=LINE('',#35169,#8220);
#6376=LINE('',#35170,#8221);
#6377=LINE('',#35174,#8222);
#6378=LINE('',#35177,#8223);
#6379=LINE('',#35178,#8224);
#6380=LINE('',#35184,#8225);
#6381=LINE('',#35186,#8226);
#6382=LINE('',#35188,#8227);
#6383=LINE('',#35189,#8228);
#6384=LINE('',#35193,#8229);
#6385=LINE('',#35196,#8230);
#6386=LINE('',#35197,#8231);
#6387=LINE('',#35203,#8232);
#6388=LINE('',#35205,#8233);
#6389=LINE('',#35207,#8234);
#6390=LINE('',#35208,#8235);
#6391=LINE('',#35212,#8236);
#6392=LINE('',#35215,#8237);
#6393=LINE('',#35216,#8238);
#6394=LINE('',#35222,#8239);
#6395=LINE('',#35224,#8240);
#6396=LINE('',#35226,#8241);
#6397=LINE('',#35227,#8242);
#6398=LINE('',#35231,#8243);
#6399=LINE('',#35234,#8244);
#6400=LINE('',#35235,#8245);
#6401=LINE('',#35241,#8246);
#6402=LINE('',#35243,#8247);
#6403=LINE('',#35245,#8248);
#6404=LINE('',#35246,#8249);
#6405=LINE('',#35250,#8250);
#6406=LINE('',#35253,#8251);
#6407=LINE('',#35254,#8252);
#6408=LINE('',#35260,#8253);
#6409=LINE('',#35262,#8254);
#6410=LINE('',#35264,#8255);
#6411=LINE('',#35265,#8256);
#6412=LINE('',#35269,#8257);
#6413=LINE('',#35272,#8258);
#6414=LINE('',#35273,#8259);
#6415=LINE('',#35279,#8260);
#6416=LINE('',#35281,#8261);
#6417=LINE('',#35283,#8262);
#6418=LINE('',#35284,#8263);
#6419=LINE('',#35288,#8264);
#6420=LINE('',#35291,#8265);
#6421=LINE('',#35292,#8266);
#6422=LINE('',#35298,#8267);
#6423=LINE('',#35300,#8268);
#6424=LINE('',#35302,#8269);
#6425=LINE('',#35303,#8270);
#6426=LINE('',#35307,#8271);
#6427=LINE('',#35310,#8272);
#6428=LINE('',#35311,#8273);
#6429=LINE('',#35317,#8274);
#6430=LINE('',#35319,#8275);
#6431=LINE('',#35321,#8276);
#6432=LINE('',#35322,#8277);
#6433=LINE('',#35326,#8278);
#6434=LINE('',#35329,#8279);
#6435=LINE('',#35330,#8280);
#6436=LINE('',#35336,#8281);
#6437=LINE('',#35338,#8282);
#6438=LINE('',#35340,#8283);
#6439=LINE('',#35341,#8284);
#6440=LINE('',#35345,#8285);
#6441=LINE('',#35348,#8286);
#6442=LINE('',#35349,#8287);
#6443=LINE('',#35355,#8288);
#6444=LINE('',#35357,#8289);
#6445=LINE('',#35359,#8290);
#6446=LINE('',#35360,#8291);
#6447=LINE('',#35364,#8292);
#6448=LINE('',#35367,#8293);
#6449=LINE('',#35368,#8294);
#6450=LINE('',#35375,#8295);
#6451=LINE('',#35380,#8296);
#6452=LINE('',#35387,#8297);
#6453=LINE('',#35392,#8298);
#6454=LINE('',#35394,#8299);
#6455=LINE('',#35402,#8300);
#6456=LINE('',#35406,#8301);
#6457=LINE('',#35411,#8302);
#6458=LINE('',#35413,#8303);
#6459=LINE('',#35415,#8304);
#6460=LINE('',#35416,#8305);
#6461=LINE('',#35419,#8306);
#6462=LINE('',#35421,#8307);
#6463=LINE('',#35422,#8308);
#6464=LINE('',#35425,#8309);
#6465=LINE('',#35427,#8310);
#6466=LINE('',#35428,#8311);
#6467=LINE('',#35431,#8312);
#6468=LINE('',#35433,#8313);
#6469=LINE('',#35434,#8314);
#6470=LINE('',#35437,#8315);
#6471=LINE('',#35439,#8316);
#6472=LINE('',#35440,#8317);
#6473=LINE('',#35442,#8318);
#6474=LINE('',#35443,#8319);
#6475=LINE('',#35448,#8320);
#6476=LINE('',#35450,#8321);
#6477=LINE('',#35452,#8322);
#6478=LINE('',#35453,#8323);
#6479=LINE('',#35457,#8324);
#6480=LINE('',#35459,#8325);
#6481=LINE('',#35460,#8326);
#6482=LINE('',#35463,#8327);
#6483=LINE('',#35464,#8328);
#6484=LINE('',#35467,#8329);
#6485=LINE('',#35468,#8330);
#6486=LINE('',#35470,#8331);
#6487=LINE('',#35476,#8332);
#8101=VECTOR('',#27284,0.4);
#8102=VECTOR('',#27285,0.4);
#8103=VECTOR('',#27292,0.4);
#8104=VECTOR('',#27295,0.4);
#8105=VECTOR('',#27298,0.4);
#8106=VECTOR('',#27301,0.4);
#8107=VECTOR('',#27304,0.4);
#8108=VECTOR('',#27307,0.4);
#8109=VECTOR('',#27310,0.4);
#8110=VECTOR('',#27313,0.4);
#8111=VECTOR('',#27316,0.4);
#8112=VECTOR('',#27319,0.352375);
#8113=VECTOR('',#27324,0.352375);
#8114=VECTOR('',#27327,0.352375);
#8115=VECTOR('',#27330,0.352375);
#8116=VECTOR('',#27333,0.352375);
#8117=VECTOR('',#27336,0.352375);
#8118=VECTOR('',#27339,0.352375);
#8119=VECTOR('',#27342,0.352375);
#8120=VECTOR('',#27345,0.352375);
#8121=VECTOR('',#27348,0.352375);
#8122=VECTOR('',#27351,0.352375);
#8123=VECTOR('',#27362,0.08);
#8124=VECTOR('',#27369,0.08);
#8125=VECTOR('',#27376,0.08);
#8126=VECTOR('',#27383,0.08);
#8127=VECTOR('',#27388,1.);
#8128=VECTOR('',#27389,1.);
#8129=VECTOR('',#27390,1.);
#8130=VECTOR('',#27391,1.);
#8131=VECTOR('',#27396,1.);
#8132=VECTOR('',#27399,1.);
#8133=VECTOR('',#27400,1.);
#8134=VECTOR('',#27407,1.);
#8135=VECTOR('',#27408,1.);
#8136=VECTOR('',#27409,1.);
#8137=VECTOR('',#27410,1.);
#8138=VECTOR('',#27415,1.);
#8139=VECTOR('',#27418,1.);
#8140=VECTOR('',#27419,1.);
#8141=VECTOR('',#27426,1.);
#8142=VECTOR('',#27427,1.);
#8143=VECTOR('',#27428,1.);
#8144=VECTOR('',#27429,1.);
#8145=VECTOR('',#27434,1.);
#8146=VECTOR('',#27437,1.);
#8147=VECTOR('',#27438,1.);
#8148=VECTOR('',#27445,1.);
#8149=VECTOR('',#27446,1.);
#8150=VECTOR('',#27447,1.);
#8151=VECTOR('',#27448,1.);
#8152=VECTOR('',#27453,1.);
#8153=VECTOR('',#27456,1.);
#8154=VECTOR('',#27457,1.);
#8155=VECTOR('',#27464,1.);
#8156=VECTOR('',#27465,1.);
#8157=VECTOR('',#27466,1.);
#8158=VECTOR('',#27467,1.);
#8159=VECTOR('',#27472,1.);
#8160=VECTOR('',#27475,1.);
#8161=VECTOR('',#27476,1.);
#8162=VECTOR('',#27483,1.);
#8163=VECTOR('',#27484,1.);
#8164=VECTOR('',#27485,1.);
#8165=VECTOR('',#27486,1.);
#8166=VECTOR('',#27491,1.);
#8167=VECTOR('',#27494,1.);
#8168=VECTOR('',#27495,1.);
#8169=VECTOR('',#27502,1.);
#8170=VECTOR('',#27503,1.);
#8171=VECTOR('',#27504,1.);
#8172=VECTOR('',#27505,1.);
#8173=VECTOR('',#27510,1.);
#8174=VECTOR('',#27513,1.);
#8175=VECTOR('',#27514,1.);
#8176=VECTOR('',#27521,1.);
#8177=VECTOR('',#27522,1.);
#8178=VECTOR('',#27523,1.);
#8179=VECTOR('',#27524,1.);
#8180=VECTOR('',#27529,1.);
#8181=VECTOR('',#27532,1.);
#8182=VECTOR('',#27533,1.);
#8183=VECTOR('',#27540,1.);
#8184=VECTOR('',#27541,1.);
#8185=VECTOR('',#27542,1.);
#8186=VECTOR('',#27543,1.);
#8187=VECTOR('',#27548,1.);
#8188=VECTOR('',#27551,1.);
#8189=VECTOR('',#27552,1.);
#8190=VECTOR('',#27559,1.);
#8191=VECTOR('',#27560,1.);
#8192=VECTOR('',#27561,1.);
#8193=VECTOR('',#27562,1.);
#8194=VECTOR('',#27567,1.);
#8195=VECTOR('',#27570,1.);
#8196=VECTOR('',#27571,1.);
#8197=VECTOR('',#27578,1.);
#8198=VECTOR('',#27579,1.);
#8199=VECTOR('',#27580,1.);
#8200=VECTOR('',#27581,1.);
#8201=VECTOR('',#27586,1.);
#8202=VECTOR('',#27589,1.);
#8203=VECTOR('',#27590,1.);
#8204=VECTOR('',#27597,1.);
#8205=VECTOR('',#27598,1.);
#8206=VECTOR('',#27599,1.);
#8207=VECTOR('',#27600,1.);
#8208=VECTOR('',#27605,1.);
#8209=VECTOR('',#27610,1.);
#8210=VECTOR('',#27611,1.);
#8211=VECTOR('',#27620,1.);
#8212=VECTOR('',#27621,1.);
#8213=VECTOR('',#27622,1.);
#8214=VECTOR('',#27623,1.);
#8215=VECTOR('',#27628,1.);
#8216=VECTOR('',#27631,1.);
#8217=VECTOR('',#27632,1.);
#8218=VECTOR('',#27639,1.);
#8219=VECTOR('',#27640,1.);
#8220=VECTOR('',#27641,1.);
#8221=VECTOR('',#27642,1.);
#8222=VECTOR('',#27647,1.);
#8223=VECTOR('',#27650,1.);
#8224=VECTOR('',#27651,1.);
#8225=VECTOR('',#27658,1.);
#8226=VECTOR('',#27659,1.);
#8227=VECTOR('',#27660,1.);
#8228=VECTOR('',#27661,1.);
#8229=VECTOR('',#27666,1.);
#8230=VECTOR('',#27669,1.);
#8231=VECTOR('',#27670,1.);
#8232=VECTOR('',#27677,1.);
#8233=VECTOR('',#27678,1.);
#8234=VECTOR('',#27679,1.);
#8235=VECTOR('',#27680,1.);
#8236=VECTOR('',#27685,1.);
#8237=VECTOR('',#27688,1.);
#8238=VECTOR('',#27689,1.);
#8239=VECTOR('',#27696,1.);
#8240=VECTOR('',#27697,1.);
#8241=VECTOR('',#27698,1.);
#8242=VECTOR('',#27699,1.);
#8243=VECTOR('',#27704,1.);
#8244=VECTOR('',#27707,1.);
#8245=VECTOR('',#27708,1.);
#8246=VECTOR('',#27715,1.);
#8247=VECTOR('',#27716,1.);
#8248=VECTOR('',#27717,1.);
#8249=VECTOR('',#27718,1.);
#8250=VECTOR('',#27723,1.);
#8251=VECTOR('',#27726,1.);
#8252=VECTOR('',#27727,1.);
#8253=VECTOR('',#27734,1.);
#8254=VECTOR('',#27735,1.);
#8255=VECTOR('',#27736,1.);
#8256=VECTOR('',#27737,1.);
#8257=VECTOR('',#27742,1.);
#8258=VECTOR('',#27745,1.);
#8259=VECTOR('',#27746,1.);
#8260=VECTOR('',#27753,1.);
#8261=VECTOR('',#27754,1.);
#8262=VECTOR('',#27755,1.);
#8263=VECTOR('',#27756,1.);
#8264=VECTOR('',#27761,1.);
#8265=VECTOR('',#27764,1.);
#8266=VECTOR('',#27765,1.);
#8267=VECTOR('',#27772,1.);
#8268=VECTOR('',#27773,1.);
#8269=VECTOR('',#27774,1.);
#8270=VECTOR('',#27775,1.);
#8271=VECTOR('',#27780,1.);
#8272=VECTOR('',#27783,1.);
#8273=VECTOR('',#27784,1.);
#8274=VECTOR('',#27791,1.);
#8275=VECTOR('',#27792,1.);
#8276=VECTOR('',#27793,1.);
#8277=VECTOR('',#27794,1.);
#8278=VECTOR('',#27799,1.);
#8279=VECTOR('',#27802,1.);
#8280=VECTOR('',#27803,1.);
#8281=VECTOR('',#27810,1.);
#8282=VECTOR('',#27811,1.);
#8283=VECTOR('',#27812,1.);
#8284=VECTOR('',#27813,1.);
#8285=VECTOR('',#27818,1.);
#8286=VECTOR('',#27821,1.);
#8287=VECTOR('',#27822,1.);
#8288=VECTOR('',#27829,1.);
#8289=VECTOR('',#27830,1.);
#8290=VECTOR('',#27831,1.);
#8291=VECTOR('',#27832,1.);
#8292=VECTOR('',#27837,1.);
#8293=VECTOR('',#27840,1.);
#8294=VECTOR('',#27841,1.);
#8295=VECTOR('',#27850,0.06);
#8296=VECTOR('',#27857,0.045);
#8297=VECTOR('',#27866,0.25);
#8298=VECTOR('',#27873,0.5);
#8299=VECTOR('',#27874,0.5);
#8300=VECTOR('',#27885,0.52);
#8301=VECTOR('',#27890,0.5);
#8302=VECTOR('',#27895,1.);
#8303=VECTOR('',#27896,1.);
#8304=VECTOR('',#27897,1.);
#8305=VECTOR('',#27898,1.);
#8306=VECTOR('',#27901,1.);
#8307=VECTOR('',#27902,1.);
#8308=VECTOR('',#27903,1.);
#8309=VECTOR('',#27906,1.);
#8310=VECTOR('',#27907,1.);
#8311=VECTOR('',#27908,1.);
#8312=VECTOR('',#27911,1.);
#8313=VECTOR('',#27912,1.);
#8314=VECTOR('',#27913,1.);
#8315=VECTOR('',#27916,1.);
#8316=VECTOR('',#27917,1.);
#8317=VECTOR('',#27918,1.);
#8318=VECTOR('',#27921,1.);
#8319=VECTOR('',#27922,1.);
#8320=VECTOR('',#27927,1.);
#8321=VECTOR('',#27928,1.);
#8322=VECTOR('',#27929,1.);
#8323=VECTOR('',#27930,1.);
#8324=VECTOR('',#27935,1.);
#8325=VECTOR('',#27936,1.);
#8326=VECTOR('',#27937,1.);
#8327=VECTOR('',#27940,1.);
#8328=VECTOR('',#27941,1.);
#8329=VECTOR('',#27944,1.);
#8330=VECTOR('',#27945,1.);
#8331=VECTOR('',#27948,1.);
#8332=VECTOR('',#27957,0.38);
#9945=VERTEX_POINT('',#33235);
#9946=VERTEX_POINT('',#33236);
#9947=VERTEX_POINT('',#33238);
#9948=VERTEX_POINT('',#33264);
#9949=VERTEX_POINT('',#33267);
#9950=VERTEX_POINT('',#33272);
#9951=VERTEX_POINT('',#33297);
#9952=VERTEX_POINT('',#33298);
#9953=VERTEX_POINT('',#33345);
#9954=VERTEX_POINT('',#33346);
#9955=VERTEX_POINT('',#33393);
#9956=VERTEX_POINT('',#33394);
#9957=VERTEX_POINT('',#33441);
#9958=VERTEX_POINT('',#33442);
#9959=VERTEX_POINT('',#33489);
#9960=VERTEX_POINT('',#33490);
#9961=VERTEX_POINT('',#33543);
#9962=VERTEX_POINT('',#33544);
#9963=VERTEX_POINT('',#33591);
#9964=VERTEX_POINT('',#33592);
#9965=VERTEX_POINT('',#33639);
#9966=VERTEX_POINT('',#33640);
#9967=VERTEX_POINT('',#33693);
#9968=VERTEX_POINT('',#33694);
#9969=VERTEX_POINT('',#33741);
#9970=VERTEX_POINT('',#33742);
#9971=VERTEX_POINT('',#33744);
#9972=VERTEX_POINT('',#33750);
#9973=VERTEX_POINT('',#33757);
#9974=VERTEX_POINT('',#33758);
#9975=VERTEX_POINT('',#33781);
#9976=VERTEX_POINT('',#33782);
#9977=VERTEX_POINT('',#33806);
#9978=VERTEX_POINT('',#33807);
#9979=VERTEX_POINT('',#33831);
#9980=VERTEX_POINT('',#33832);
#9981=VERTEX_POINT('',#33855);
#9982=VERTEX_POINT('',#33856);
#9983=VERTEX_POINT('',#33880);
#9984=VERTEX_POINT('',#33881);
#9985=VERTEX_POINT('',#33905);
#9986=VERTEX_POINT('',#33906);
#9987=VERTEX_POINT('',#33929);
#9988=VERTEX_POINT('',#33930);
#9989=VERTEX_POINT('',#33955);
#9990=VERTEX_POINT('',#33956);
#9991=VERTEX_POINT('',#33979);
#9992=VERTEX_POINT('',#33980);
#9993=VERTEX_POINT('',#34295);
#9994=VERTEX_POINT('',#34373);
#9995=VERTEX_POINT('',#34447);
#9996=VERTEX_POINT('',#34809);
#9997=VERTEX_POINT('',#34888);
#9998=VERTEX_POINT('',#34890);
#9999=VERTEX_POINT('',#34894);
#10000=VERTEX_POINT('',#34896);
#10001=VERTEX_POINT('',#34900);
#10002=VERTEX_POINT('',#34902);
#10003=VERTEX_POINT('',#34906);
#10004=VERTEX_POINT('',#34908);
#10005=VERTEX_POINT('',#34912);
#10006=VERTEX_POINT('',#34913);
#10007=VERTEX_POINT('',#34915);
#10008=VERTEX_POINT('',#34917);
#10009=VERTEX_POINT('',#34921);
#10010=VERTEX_POINT('',#34925);
#10011=VERTEX_POINT('',#34931);
#10012=VERTEX_POINT('',#34932);
#10013=VERTEX_POINT('',#34934);
#10014=VERTEX_POINT('',#34936);
#10015=VERTEX_POINT('',#34940);
#10016=VERTEX_POINT('',#34944);
#10017=VERTEX_POINT('',#34950);
#10018=VERTEX_POINT('',#34951);
#10019=VERTEX_POINT('',#34953);
#10020=VERTEX_POINT('',#34955);
#10021=VERTEX_POINT('',#34959);
#10022=VERTEX_POINT('',#34963);
#10023=VERTEX_POINT('',#34969);
#10024=VERTEX_POINT('',#34970);
#10025=VERTEX_POINT('',#34972);
#10026=VERTEX_POINT('',#34974);
#10027=VERTEX_POINT('',#34978);
#10028=VERTEX_POINT('',#34982);
#10029=VERTEX_POINT('',#34988);
#10030=VERTEX_POINT('',#34989);
#10031=VERTEX_POINT('',#34991);
#10032=VERTEX_POINT('',#34993);
#10033=VERTEX_POINT('',#34997);
#10034=VERTEX_POINT('',#35001);
#10035=VERTEX_POINT('',#35007);
#10036=VERTEX_POINT('',#35008);
#10037=VERTEX_POINT('',#35010);
#10038=VERTEX_POINT('',#35012);
#10039=VERTEX_POINT('',#35016);
#10040=VERTEX_POINT('',#35020);
#10041=VERTEX_POINT('',#35026);
#10042=VERTEX_POINT('',#35027);
#10043=VERTEX_POINT('',#35029);
#10044=VERTEX_POINT('',#35031);
#10045=VERTEX_POINT('',#35035);
#10046=VERTEX_POINT('',#35039);
#10047=VERTEX_POINT('',#35045);
#10048=VERTEX_POINT('',#35046);
#10049=VERTEX_POINT('',#35048);
#10050=VERTEX_POINT('',#35050);
#10051=VERTEX_POINT('',#35054);
#10052=VERTEX_POINT('',#35058);
#10053=VERTEX_POINT('',#35064);
#10054=VERTEX_POINT('',#35065);
#10055=VERTEX_POINT('',#35067);
#10056=VERTEX_POINT('',#35069);
#10057=VERTEX_POINT('',#35073);
#10058=VERTEX_POINT('',#35077);
#10059=VERTEX_POINT('',#35083);
#10060=VERTEX_POINT('',#35084);
#10061=VERTEX_POINT('',#35086);
#10062=VERTEX_POINT('',#35088);
#10063=VERTEX_POINT('',#35092);
#10064=VERTEX_POINT('',#35096);
#10065=VERTEX_POINT('',#35102);
#10066=VERTEX_POINT('',#35103);
#10067=VERTEX_POINT('',#35105);
#10068=VERTEX_POINT('',#35107);
#10069=VERTEX_POINT('',#35111);
#10070=VERTEX_POINT('',#35115);
#10071=VERTEX_POINT('',#35121);
#10072=VERTEX_POINT('',#35122);
#10073=VERTEX_POINT('',#35124);
#10074=VERTEX_POINT('',#35126);
#10075=VERTEX_POINT('',#35130);
#10076=VERTEX_POINT('',#35132);
#10077=VERTEX_POINT('',#35136);
#10078=VERTEX_POINT('',#35140);
#10079=VERTEX_POINT('',#35144);
#10080=VERTEX_POINT('',#35145);
#10081=VERTEX_POINT('',#35147);
#10082=VERTEX_POINT('',#35149);
#10083=VERTEX_POINT('',#35153);
#10084=VERTEX_POINT('',#35157);
#10085=VERTEX_POINT('',#35163);
#10086=VERTEX_POINT('',#35164);
#10087=VERTEX_POINT('',#35166);
#10088=VERTEX_POINT('',#35168);
#10089=VERTEX_POINT('',#35172);
#10090=VERTEX_POINT('',#35176);
#10091=VERTEX_POINT('',#35182);
#10092=VERTEX_POINT('',#35183);
#10093=VERTEX_POINT('',#35185);
#10094=VERTEX_POINT('',#35187);
#10095=VERTEX_POINT('',#35191);
#10096=VERTEX_POINT('',#35195);
#10097=VERTEX_POINT('',#35201);
#10098=VERTEX_POINT('',#35202);
#10099=VERTEX_POINT('',#35204);
#10100=VERTEX_POINT('',#35206);
#10101=VERTEX_POINT('',#35210);
#10102=VERTEX_POINT('',#35214);
#10103=VERTEX_POINT('',#35220);
#10104=VERTEX_POINT('',#35221);
#10105=VERTEX_POINT('',#35223);
#10106=VERTEX_POINT('',#35225);
#10107=VERTEX_POINT('',#35229);
#10108=VERTEX_POINT('',#35233);
#10109=VERTEX_POINT('',#35239);
#10110=VERTEX_POINT('',#35240);
#10111=VERTEX_POINT('',#35242);
#10112=VERTEX_POINT('',#35244);
#10113=VERTEX_POINT('',#35248);
#10114=VERTEX_POINT('',#35252);
#10115=VERTEX_POINT('',#35258);
#10116=VERTEX_POINT('',#35259);
#10117=VERTEX_POINT('',#35261);
#10118=VERTEX_POINT('',#35263);
#10119=VERTEX_POINT('',#35267);
#10120=VERTEX_POINT('',#35271);
#10121=VERTEX_POINT('',#35277);
#10122=VERTEX_POINT('',#35278);
#10123=VERTEX_POINT('',#35280);
#10124=VERTEX_POINT('',#35282);
#10125=VERTEX_POINT('',#35286);
#10126=VERTEX_POINT('',#35290);
#10127=VERTEX_POINT('',#35296);
#10128=VERTEX_POINT('',#35297);
#10129=VERTEX_POINT('',#35299);
#10130=VERTEX_POINT('',#35301);
#10131=VERTEX_POINT('',#35305);
#10132=VERTEX_POINT('',#35309);
#10133=VERTEX_POINT('',#35315);
#10134=VERTEX_POINT('',#35316);
#10135=VERTEX_POINT('',#35318);
#10136=VERTEX_POINT('',#35320);
#10137=VERTEX_POINT('',#35324);
#10138=VERTEX_POINT('',#35328);
#10139=VERTEX_POINT('',#35334);
#10140=VERTEX_POINT('',#35335);
#10141=VERTEX_POINT('',#35337);
#10142=VERTEX_POINT('',#35339);
#10143=VERTEX_POINT('',#35343);
#10144=VERTEX_POINT('',#35347);
#10145=VERTEX_POINT('',#35353);
#10146=VERTEX_POINT('',#35354);
#10147=VERTEX_POINT('',#35356);
#10148=VERTEX_POINT('',#35358);
#10149=VERTEX_POINT('',#35362);
#10150=VERTEX_POINT('',#35366);
#10151=VERTEX_POINT('',#35372);
#10152=VERTEX_POINT('',#35374);
#10153=VERTEX_POINT('',#35378);
#10154=VERTEX_POINT('',#35383);
#10155=VERTEX_POINT('',#35386);
#10156=VERTEX_POINT('',#35390);
#10157=VERTEX_POINT('',#35393);
#10158=VERTEX_POINT('',#35397);
#10159=VERTEX_POINT('',#35400);
#10160=VERTEX_POINT('',#35404);
#10161=VERTEX_POINT('',#35409);
#10162=VERTEX_POINT('',#35410);
#10163=VERTEX_POINT('',#35412);
#10164=VERTEX_POINT('',#35414);
#10165=VERTEX_POINT('',#35418);
#10166=VERTEX_POINT('',#35420);
#10167=VERTEX_POINT('',#35424);
#10168=VERTEX_POINT('',#35426);
#10169=VERTEX_POINT('',#35430);
#10170=VERTEX_POINT('',#35432);
#10171=VERTEX_POINT('',#35436);
#10172=VERTEX_POINT('',#35438);
#10173=VERTEX_POINT('',#35446);
#10174=VERTEX_POINT('',#35447);
#10175=VERTEX_POINT('',#35449);
#10176=VERTEX_POINT('',#35451);
#10177=VERTEX_POINT('',#35456);
#10178=VERTEX_POINT('',#35458);
#10179=VERTEX_POINT('',#35462);
#10180=VERTEX_POINT('',#35466);
#10181=VERTEX_POINT('',#35473);
#12401=EDGE_CURVE('',#9945,#9946,#6256,.T.);
#12402=EDGE_CURVE('',#9945,#9947,#373,.T.);
#12403=EDGE_CURVE('',#9947,#9948,#6257,.T.);
#12404=EDGE_CURVE('',#9948,#9948,#5349,.T.);
#12405=EDGE_CURVE('',#9947,#9949,#374,.T.);
#12406=EDGE_CURVE('',#9949,#9950,#5350,.T.);
#12407=EDGE_CURVE('',#9950,#9946,#375,.T.);
#12408=EDGE_CURVE('',#9951,#9952,#6258,.T.);
#12409=EDGE_CURVE('',#9951,#9945,#376,.T.);
#12410=EDGE_CURVE('',#9946,#9952,#377,.T.);
#12411=EDGE_CURVE('',#9953,#9954,#6259,.T.);
#12412=EDGE_CURVE('',#9953,#9951,#378,.T.);
#12413=EDGE_CURVE('',#9952,#9954,#379,.T.);
#12414=EDGE_CURVE('',#9955,#9956,#6260,.T.);
#12415=EDGE_CURVE('',#9955,#9953,#380,.T.);
#12416=EDGE_CURVE('',#9954,#9956,#381,.T.);
#12417=EDGE_CURVE('',#9957,#9958,#6261,.T.);
#12418=EDGE_CURVE('',#9957,#9955,#382,.T.);
#12419=EDGE_CURVE('',#9956,#9958,#383,.T.);
#12420=EDGE_CURVE('',#9959,#9960,#6262,.T.);
#12421=EDGE_CURVE('',#9959,#9957,#384,.T.);
#12422=EDGE_CURVE('',#9958,#9960,#385,.T.);
#12423=EDGE_CURVE('',#9961,#9962,#6263,.T.);
#12424=EDGE_CURVE('',#9961,#9959,#386,.T.);
#12425=EDGE_CURVE('',#9960,#9962,#387,.T.);
#12426=EDGE_CURVE('',#9963,#9964,#6264,.T.);
#12427=EDGE_CURVE('',#9963,#9961,#388,.T.);
#12428=EDGE_CURVE('',#9962,#9964,#389,.T.);
#12429=EDGE_CURVE('',#9965,#9966,#6265,.T.);
#12430=EDGE_CURVE('',#9965,#9963,#390,.T.);
#12431=EDGE_CURVE('',#9964,#9966,#391,.T.);
#12432=EDGE_CURVE('',#9967,#9968,#6266,.T.);
#12433=EDGE_CURVE('',#9967,#9965,#392,.T.);
#12434=EDGE_CURVE('',#9966,#9968,#393,.T.);
#12435=EDGE_CURVE('',#9969,#9970,#6267,.T.);
#12436=EDGE_CURVE('',#9969,#9971,#394,.T.);
#12437=EDGE_CURVE('',#9972,#9971,#5351,.T.);
#12438=EDGE_CURVE('',#9970,#9972,#395,.T.);
#12439=EDGE_CURVE('',#9973,#9974,#6268,.T.);
#12440=EDGE_CURVE('',#9973,#9969,#396,.T.);
#12441=EDGE_CURVE('',#9974,#9970,#397,.T.);
#12442=EDGE_CURVE('',#9975,#9976,#6269,.T.);
#12443=EDGE_CURVE('',#9975,#9973,#398,.T.);
#12444=EDGE_CURVE('',#9976,#9974,#399,.T.);
#12445=EDGE_CURVE('',#9977,#9978,#6270,.T.);
#12446=EDGE_CURVE('',#9977,#9975,#400,.T.);
#12447=EDGE_CURVE('',#9978,#9976,#401,.T.);
#12448=EDGE_CURVE('',#9979,#9980,#6271,.T.);
#12449=EDGE_CURVE('',#9979,#9977,#402,.T.);
#12450=EDGE_CURVE('',#9980,#9978,#403,.T.);
#12451=EDGE_CURVE('',#9981,#9982,#6272,.T.);
#12452=EDGE_CURVE('',#9981,#9979,#404,.T.);
#12453=EDGE_CURVE('',#9982,#9980,#405,.T.);
#12454=EDGE_CURVE('',#9983,#9984,#6273,.T.);
#12455=EDGE_CURVE('',#9983,#9981,#406,.T.);
#12456=EDGE_CURVE('',#9984,#9982,#407,.T.);
#12457=EDGE_CURVE('',#9985,#9986,#6274,.T.);
#12458=EDGE_CURVE('',#9985,#9983,#408,.T.);
#12459=EDGE_CURVE('',#9986,#9984,#409,.T.);
#12460=EDGE_CURVE('',#9987,#9988,#6275,.T.);
#12461=EDGE_CURVE('',#9987,#9985,#410,.T.);
#12462=EDGE_CURVE('',#9988,#9986,#411,.T.);
#12463=EDGE_CURVE('',#9989,#9990,#6276,.T.);
#12464=EDGE_CURVE('',#9989,#9987,#412,.T.);
#12465=EDGE_CURVE('',#9990,#9988,#413,.T.);
#12466=EDGE_CURVE('',#9991,#9992,#6277,.T.);
#12467=EDGE_CURVE('',#9991,#9989,#414,.T.);
#12468=EDGE_CURVE('',#9992,#9990,#415,.T.);
#12469=EDGE_CURVE('',#9993,#9972,#416,.T.);
#12470=EDGE_CURVE('',#9968,#9993,#417,.T.);
#12471=EDGE_CURVE('',#9994,#9950,#418,.T.);
#12472=EDGE_CURVE('',#9994,#9992,#419,.T.);
#12473=EDGE_CURVE('',#9949,#9995,#420,.T.);
#12474=EDGE_CURVE('',#9995,#9994,#5352,.T.);
#12475=EDGE_CURVE('',#9995,#9991,#421,.T.);
#12476=EDGE_CURVE('',#9971,#9996,#422,.T.);
#12477=EDGE_CURVE('',#9996,#9967,#423,.T.);
#12478=EDGE_CURVE('',#9997,#9997,#5353,.T.);
#12479=EDGE_CURVE('',#9997,#9998,#6278,.T.);
#12480=EDGE_CURVE('',#9998,#9998,#5354,.T.);
#12481=EDGE_CURVE('',#9999,#9999,#5355,.T.);
#12482=EDGE_CURVE('',#9999,#10000,#6279,.T.);
#12483=EDGE_CURVE('',#10000,#10000,#5356,.T.);
#12484=EDGE_CURVE('',#10001,#10001,#5357,.T.);
#12485=EDGE_CURVE('',#10001,#10002,#6280,.T.);
#12486=EDGE_CURVE('',#10002,#10002,#5358,.T.);
#12487=EDGE_CURVE('',#10003,#10003,#5359,.T.);
#12488=EDGE_CURVE('',#10003,#10004,#6281,.T.);
#12489=EDGE_CURVE('',#10004,#10004,#5360,.T.);
#12490=EDGE_CURVE('',#10005,#10006,#6282,.T.);
#12491=EDGE_CURVE('',#10007,#10005,#6283,.T.);
#12492=EDGE_CURVE('',#10007,#10008,#6284,.T.);
#12493=EDGE_CURVE('',#10008,#10006,#6285,.T.);
#12494=EDGE_CURVE('',#10006,#10009,#5361,.T.);
#12495=EDGE_CURVE('',#10009,#10008,#6286,.T.);
#12496=EDGE_CURVE('',#10009,#10010,#6287,.T.);
#12497=EDGE_CURVE('',#10010,#10007,#6288,.T.);
#12498=EDGE_CURVE('',#10010,#10005,#5362,.T.);
#12499=EDGE_CURVE('',#10011,#10012,#6289,.T.);
#12500=EDGE_CURVE('',#10013,#10011,#6290,.T.);
#12501=EDGE_CURVE('',#10013,#10014,#6291,.T.);
#12502=EDGE_CURVE('',#10014,#10012,#6292,.T.);
#12503=EDGE_CURVE('',#10012,#10015,#5363,.T.);
#12504=EDGE_CURVE('',#10015,#10014,#6293,.T.);
#12505=EDGE_CURVE('',#10015,#10016,#6294,.T.);
#12506=EDGE_CURVE('',#10016,#10013,#6295,.T.);
#12507=EDGE_CURVE('',#10016,#10011,#5364,.T.);
#12508=EDGE_CURVE('',#10017,#10018,#6296,.T.);
#12509=EDGE_CURVE('',#10019,#10017,#6297,.T.);
#12510=EDGE_CURVE('',#10019,#10020,#6298,.T.);
#12511=EDGE_CURVE('',#10020,#10018,#6299,.T.);
#12512=EDGE_CURVE('',#10018,#10021,#5365,.T.);
#12513=EDGE_CURVE('',#10021,#10020,#6300,.T.);
#12514=EDGE_CURVE('',#10021,#10022,#6301,.T.);
#12515=EDGE_CURVE('',#10022,#10019,#6302,.T.);
#12516=EDGE_CURVE('',#10022,#10017,#5366,.T.);
#12517=EDGE_CURVE('',#10023,#10024,#6303,.T.);
#12518=EDGE_CURVE('',#10025,#10023,#6304,.T.);
#12519=EDGE_CURVE('',#10025,#10026,#6305,.T.);
#12520=EDGE_CURVE('',#10026,#10024,#6306,.T.);
#12521=EDGE_CURVE('',#10024,#10027,#5367,.T.);
#12522=EDGE_CURVE('',#10027,#10026,#6307,.T.);
#12523=EDGE_CURVE('',#10027,#10028,#6308,.T.);
#12524=EDGE_CURVE('',#10028,#10025,#6309,.T.);
#12525=EDGE_CURVE('',#10028,#10023,#5368,.T.);
#12526=EDGE_CURVE('',#10029,#10030,#6310,.T.);
#12527=EDGE_CURVE('',#10031,#10029,#6311,.T.);
#12528=EDGE_CURVE('',#10031,#10032,#6312,.T.);
#12529=EDGE_CURVE('',#10032,#10030,#6313,.T.);
#12530=EDGE_CURVE('',#10030,#10033,#5369,.T.);
#12531=EDGE_CURVE('',#10033,#10032,#6314,.T.);
#12532=EDGE_CURVE('',#10033,#10034,#6315,.T.);
#12533=EDGE_CURVE('',#10034,#10031,#6316,.T.);
#12534=EDGE_CURVE('',#10034,#10029,#5370,.T.);
#12535=EDGE_CURVE('',#10035,#10036,#6317,.T.);
#12536=EDGE_CURVE('',#10037,#10035,#6318,.T.);
#12537=EDGE_CURVE('',#10037,#10038,#6319,.T.);
#12538=EDGE_CURVE('',#10038,#10036,#6320,.T.);
#12539=EDGE_CURVE('',#10036,#10039,#5371,.T.);
#12540=EDGE_CURVE('',#10039,#10038,#6321,.T.);
#12541=EDGE_CURVE('',#10039,#10040,#6322,.T.);
#12542=EDGE_CURVE('',#10040,#10037,#6323,.T.);
#12543=EDGE_CURVE('',#10040,#10035,#5372,.T.);
#12544=EDGE_CURVE('',#10041,#10042,#6324,.T.);
#12545=EDGE_CURVE('',#10043,#10041,#6325,.T.);
#12546=EDGE_CURVE('',#10043,#10044,#6326,.T.);
#12547=EDGE_CURVE('',#10044,#10042,#6327,.T.);
#12548=EDGE_CURVE('',#10042,#10045,#5373,.T.);
#12549=EDGE_CURVE('',#10045,#10044,#6328,.T.);
#12550=EDGE_CURVE('',#10045,#10046,#6329,.T.);
#12551=EDGE_CURVE('',#10046,#10043,#6330,.T.);
#12552=EDGE_CURVE('',#10046,#10041,#5374,.T.);
#12553=EDGE_CURVE('',#10047,#10048,#6331,.T.);
#12554=EDGE_CURVE('',#10049,#10047,#6332,.T.);
#12555=EDGE_CURVE('',#10049,#10050,#6333,.T.);
#12556=EDGE_CURVE('',#10050,#10048,#6334,.T.);
#12557=EDGE_CURVE('',#10048,#10051,#5375,.T.);
#12558=EDGE_CURVE('',#10051,#10050,#6335,.T.);
#12559=EDGE_CURVE('',#10051,#10052,#6336,.T.);
#12560=EDGE_CURVE('',#10052,#10049,#6337,.T.);
#12561=EDGE_CURVE('',#10052,#10047,#5376,.T.);
#12562=EDGE_CURVE('',#10053,#10054,#6338,.T.);
#12563=EDGE_CURVE('',#10055,#10053,#6339,.T.);
#12564=EDGE_CURVE('',#10055,#10056,#6340,.T.);
#12565=EDGE_CURVE('',#10056,#10054,#6341,.T.);
#12566=EDGE_CURVE('',#10054,#10057,#5377,.T.);
#12567=EDGE_CURVE('',#10057,#10056,#6342,.T.);
#12568=EDGE_CURVE('',#10057,#10058,#6343,.T.);
#12569=EDGE_CURVE('',#10058,#10055,#6344,.T.);
#12570=EDGE_CURVE('',#10058,#10053,#5378,.T.);
#12571=EDGE_CURVE('',#10059,#10060,#6345,.T.);
#12572=EDGE_CURVE('',#10061,#10059,#6346,.T.);
#12573=EDGE_CURVE('',#10061,#10062,#6347,.T.);
#12574=EDGE_CURVE('',#10062,#10060,#6348,.T.);
#12575=EDGE_CURVE('',#10060,#10063,#5379,.T.);
#12576=EDGE_CURVE('',#10063,#10062,#6349,.T.);
#12577=EDGE_CURVE('',#10063,#10064,#6350,.T.);
#12578=EDGE_CURVE('',#10064,#10061,#6351,.T.);
#12579=EDGE_CURVE('',#10064,#10059,#5380,.T.);
#12580=EDGE_CURVE('',#10065,#10066,#6352,.T.);
#12581=EDGE_CURVE('',#10067,#10065,#6353,.T.);
#12582=EDGE_CURVE('',#10067,#10068,#6354,.T.);
#12583=EDGE_CURVE('',#10068,#10066,#6355,.T.);
#12584=EDGE_CURVE('',#10066,#10069,#5381,.T.);
#12585=EDGE_CURVE('',#10069,#10068,#6356,.T.);
#12586=EDGE_CURVE('',#10069,#10070,#6357,.T.);
#12587=EDGE_CURVE('',#10070,#10067,#6358,.T.);
#12588=EDGE_CURVE('',#10070,#10065,#5382,.T.);
#12589=EDGE_CURVE('',#10071,#10072,#6359,.T.);
#12590=EDGE_CURVE('',#10073,#10071,#6360,.T.);
#12591=EDGE_CURVE('',#10073,#10074,#6361,.T.);
#12592=EDGE_CURVE('',#10074,#10072,#6362,.T.);
#12593=EDGE_CURVE('',#10072,#10075,#5383,.T.);
#12594=EDGE_CURVE('',#10076,#10074,#6363,.T.);
#12595=EDGE_CURVE('',#10075,#10076,#5384,.T.);
#12596=EDGE_CURVE('',#10076,#10077,#6364,.T.);
#12597=EDGE_CURVE('',#10077,#10073,#6365,.T.);
#12598=EDGE_CURVE('',#10077,#10078,#5385,.T.);
#12599=EDGE_CURVE('',#10078,#10071,#5386,.T.);
#12600=EDGE_CURVE('',#10079,#10080,#6366,.T.);
#12601=EDGE_CURVE('',#10081,#10079,#6367,.T.);
#12602=EDGE_CURVE('',#10081,#10082,#6368,.T.);
#12603=EDGE_CURVE('',#10082,#10080,#6369,.T.);
#12604=EDGE_CURVE('',#10080,#10083,#5387,.T.);
#12605=EDGE_CURVE('',#10083,#10082,#6370,.T.);
#12606=EDGE_CURVE('',#10083,#10084,#6371,.T.);
#12607=EDGE_CURVE('',#10084,#10081,#6372,.T.);
#12608=EDGE_CURVE('',#10084,#10079,#5388,.T.);
#12609=EDGE_CURVE('',#10085,#10086,#6373,.T.);
#12610=EDGE_CURVE('',#10087,#10085,#6374,.T.);
#12611=EDGE_CURVE('',#10087,#10088,#6375,.T.);
#12612=EDGE_CURVE('',#10088,#10086,#6376,.T.);
#12613=EDGE_CURVE('',#10086,#10089,#5389,.T.);
#12614=EDGE_CURVE('',#10089,#10088,#6377,.T.);
#12615=EDGE_CURVE('',#10089,#10090,#6378,.T.);
#12616=EDGE_CURVE('',#10090,#10087,#6379,.T.);
#12617=EDGE_CURVE('',#10090,#10085,#5390,.T.);
#12618=EDGE_CURVE('',#10091,#10092,#6380,.T.);
#12619=EDGE_CURVE('',#10093,#10091,#6381,.T.);
#12620=EDGE_CURVE('',#10093,#10094,#6382,.T.);
#12621=EDGE_CURVE('',#10094,#10092,#6383,.T.);
#12622=EDGE_CURVE('',#10092,#10095,#5391,.T.);
#12623=EDGE_CURVE('',#10095,#10094,#6384,.T.);
#12624=EDGE_CURVE('',#10095,#10096,#6385,.T.);
#12625=EDGE_CURVE('',#10096,#10093,#6386,.T.);
#12626=EDGE_CURVE('',#10096,#10091,#5392,.T.);
#12627=EDGE_CURVE('',#10097,#10098,#6387,.T.);
#12628=EDGE_CURVE('',#10099,#10097,#6388,.T.);
#12629=EDGE_CURVE('',#10099,#10100,#6389,.T.);
#12630=EDGE_CURVE('',#10100,#10098,#6390,.T.);
#12631=EDGE_CURVE('',#10098,#10101,#5393,.T.);
#12632=EDGE_CURVE('',#10101,#10100,#6391,.T.);
#12633=EDGE_CURVE('',#10101,#10102,#6392,.T.);
#12634=EDGE_CURVE('',#10102,#10099,#6393,.T.);
#12635=EDGE_CURVE('',#10102,#10097,#5394,.T.);
#12636=EDGE_CURVE('',#10103,#10104,#6394,.T.);
#12637=EDGE_CURVE('',#10105,#10103,#6395,.T.);
#12638=EDGE_CURVE('',#10105,#10106,#6396,.T.);
#12639=EDGE_CURVE('',#10106,#10104,#6397,.T.);
#12640=EDGE_CURVE('',#10104,#10107,#5395,.T.);
#12641=EDGE_CURVE('',#10107,#10106,#6398,.T.);
#12642=EDGE_CURVE('',#10107,#10108,#6399,.T.);
#12643=EDGE_CURVE('',#10108,#10105,#6400,.T.);
#12644=EDGE_CURVE('',#10108,#10103,#5396,.T.);
#12645=EDGE_CURVE('',#10109,#10110,#6401,.T.);
#12646=EDGE_CURVE('',#10111,#10109,#6402,.T.);
#12647=EDGE_CURVE('',#10111,#10112,#6403,.T.);
#12648=EDGE_CURVE('',#10112,#10110,#6404,.T.);
#12649=EDGE_CURVE('',#10110,#10113,#5397,.T.);
#12650=EDGE_CURVE('',#10113,#10112,#6405,.T.);
#12651=EDGE_CURVE('',#10113,#10114,#6406,.T.);
#12652=EDGE_CURVE('',#10114,#10111,#6407,.T.);
#12653=EDGE_CURVE('',#10114,#10109,#5398,.T.);
#12654=EDGE_CURVE('',#10115,#10116,#6408,.T.);
#12655=EDGE_CURVE('',#10117,#10115,#6409,.T.);
#12656=EDGE_CURVE('',#10117,#10118,#6410,.T.);
#12657=EDGE_CURVE('',#10118,#10116,#6411,.T.);
#12658=EDGE_CURVE('',#10116,#10119,#5399,.T.);
#12659=EDGE_CURVE('',#10119,#10118,#6412,.T.);
#12660=EDGE_CURVE('',#10119,#10120,#6413,.T.);
#12661=EDGE_CURVE('',#10120,#10117,#6414,.T.);
#12662=EDGE_CURVE('',#10120,#10115,#5400,.T.);
#12663=EDGE_CURVE('',#10121,#10122,#6415,.T.);
#12664=EDGE_CURVE('',#10123,#10121,#6416,.T.);
#12665=EDGE_CURVE('',#10123,#10124,#6417,.T.);
#12666=EDGE_CURVE('',#10124,#10122,#6418,.T.);
#12667=EDGE_CURVE('',#10122,#10125,#5401,.T.);
#12668=EDGE_CURVE('',#10125,#10124,#6419,.T.);
#12669=EDGE_CURVE('',#10125,#10126,#6420,.T.);
#12670=EDGE_CURVE('',#10126,#10123,#6421,.T.);
#12671=EDGE_CURVE('',#10126,#10121,#5402,.T.);
#12672=EDGE_CURVE('',#10127,#10128,#6422,.T.);
#12673=EDGE_CURVE('',#10129,#10127,#6423,.T.);
#12674=EDGE_CURVE('',#10129,#10130,#6424,.T.);
#12675=EDGE_CURVE('',#10130,#10128,#6425,.T.);
#12676=EDGE_CURVE('',#10128,#10131,#5403,.T.);
#12677=EDGE_CURVE('',#10131,#10130,#6426,.T.);
#12678=EDGE_CURVE('',#10131,#10132,#6427,.T.);
#12679=EDGE_CURVE('',#10132,#10129,#6428,.T.);
#12680=EDGE_CURVE('',#10132,#10127,#5404,.T.);
#12681=EDGE_CURVE('',#10133,#10134,#6429,.T.);
#12682=EDGE_CURVE('',#10135,#10133,#6430,.T.);
#12683=EDGE_CURVE('',#10135,#10136,#6431,.T.);
#12684=EDGE_CURVE('',#10136,#10134,#6432,.T.);
#12685=EDGE_CURVE('',#10134,#10137,#5405,.T.);
#12686=EDGE_CURVE('',#10137,#10136,#6433,.T.);
#12687=EDGE_CURVE('',#10137,#10138,#6434,.T.);
#12688=EDGE_CURVE('',#10138,#10135,#6435,.T.);
#12689=EDGE_CURVE('',#10138,#10133,#5406,.T.);
#12690=EDGE_CURVE('',#10139,#10140,#6436,.T.);
#12691=EDGE_CURVE('',#10141,#10139,#6437,.T.);
#12692=EDGE_CURVE('',#10141,#10142,#6438,.T.);
#12693=EDGE_CURVE('',#10142,#10140,#6439,.T.);
#12694=EDGE_CURVE('',#10140,#10143,#5407,.T.);
#12695=EDGE_CURVE('',#10143,#10142,#6440,.T.);
#12696=EDGE_CURVE('',#10143,#10144,#6441,.T.);
#12697=EDGE_CURVE('',#10144,#10141,#6442,.T.);
#12698=EDGE_CURVE('',#10144,#10139,#5408,.T.);
#12699=EDGE_CURVE('',#10145,#10146,#6443,.T.);
#12700=EDGE_CURVE('',#10147,#10145,#6444,.T.);
#12701=EDGE_CURVE('',#10147,#10148,#6445,.T.);
#12702=EDGE_CURVE('',#10148,#10146,#6446,.T.);
#12703=EDGE_CURVE('',#10146,#10149,#5409,.T.);
#12704=EDGE_CURVE('',#10149,#10148,#6447,.T.);
#12705=EDGE_CURVE('',#10149,#10150,#6448,.T.);
#12706=EDGE_CURVE('',#10150,#10147,#6449,.T.);
#12707=EDGE_CURVE('',#10150,#10145,#5410,.T.);
#12708=EDGE_CURVE('',#10151,#10151,#5411,.T.);
#12709=EDGE_CURVE('',#10151,#10152,#6450,.T.);
#12710=EDGE_CURVE('',#10152,#10152,#5412,.T.);
#12711=EDGE_CURVE('',#10153,#10153,#5413,.T.);
#12712=EDGE_CURVE('',#10153,#10151,#6451,.T.);
#12713=EDGE_CURVE('',#10154,#10154,#5414,.T.);
#12714=EDGE_CURVE('',#10154,#10155,#6452,.T.);
#12715=EDGE_CURVE('',#10155,#10155,#5415,.T.);
#12716=EDGE_CURVE('',#10156,#10156,#5416,.T.);
#12717=EDGE_CURVE('',#10156,#10075,#6453,.T.);
#12718=EDGE_CURVE('',#10078,#10157,#6454,.T.);
#12719=EDGE_CURVE('',#10157,#10157,#5417,.T.);
#12720=EDGE_CURVE('',#10158,#10158,#5418,.T.);
#12721=EDGE_CURVE('',#10159,#10159,#5419,.T.);
#12722=EDGE_CURVE('',#10159,#10158,#6455,.T.);
#12723=EDGE_CURVE('',#10160,#10160,#5420,.T.);
#12724=EDGE_CURVE('',#10160,#10159,#6456,.T.);
#12725=EDGE_CURVE('',#10161,#10162,#6457,.T.);
#12726=EDGE_CURVE('',#10161,#10163,#6458,.T.);
#12727=EDGE_CURVE('',#10164,#10163,#6459,.T.);
#12728=EDGE_CURVE('',#10162,#10164,#6460,.T.);
#12729=EDGE_CURVE('',#10162,#10165,#6461,.T.);
#12730=EDGE_CURVE('',#10166,#10164,#6462,.T.);
#12731=EDGE_CURVE('',#10165,#10166,#6463,.T.);
#12732=EDGE_CURVE('',#10165,#10167,#6464,.T.);
#12733=EDGE_CURVE('',#10168,#10166,#6465,.T.);
#12734=EDGE_CURVE('',#10167,#10168,#6466,.T.);
#12735=EDGE_CURVE('',#10167,#10169,#6467,.T.);
#12736=EDGE_CURVE('',#10170,#10168,#6468,.T.);
#12737=EDGE_CURVE('',#10169,#10170,#6469,.T.);
#12738=EDGE_CURVE('',#10169,#10171,#6470,.T.);
#12739=EDGE_CURVE('',#10172,#10170,#6471,.T.);
#12740=EDGE_CURVE('',#10171,#10172,#6472,.T.);
#12741=EDGE_CURVE('',#10171,#10161,#6473,.T.);
#12742=EDGE_CURVE('',#10163,#10172,#6474,.T.);
#12743=EDGE_CURVE('',#10173,#10174,#6475,.T.);
#12744=EDGE_CURVE('',#10175,#10173,#6476,.T.);
#12745=EDGE_CURVE('',#10176,#10175,#6477,.T.);
#12746=EDGE_CURVE('',#10174,#10176,#6478,.T.);
#12747=EDGE_CURVE('',#9996,#9993,#5421,.F.);
#12748=EDGE_CURVE('',#10173,#10177,#6479,.T.);
#12749=EDGE_CURVE('',#10178,#10177,#6480,.T.);
#12750=EDGE_CURVE('',#10175,#10178,#6481,.T.);
#12751=EDGE_CURVE('',#10179,#10178,#6482,.T.);
#12752=EDGE_CURVE('',#10176,#10179,#6483,.T.);
#12753=EDGE_CURVE('',#10180,#10179,#6484,.T.);
#12754=EDGE_CURVE('',#10174,#10180,#6485,.T.);
#12755=EDGE_CURVE('',#10177,#10180,#6486,.T.);
#12756=EDGE_CURVE('',#10181,#10181,#5422,.T.);
#12757=EDGE_CURVE('',#9948,#10181,#6487,.T.);
#16447=ORIENTED_EDGE('',*,*,#12401,.F.);
#16448=ORIENTED_EDGE('',*,*,#12402,.T.);
#16449=ORIENTED_EDGE('',*,*,#12403,.T.);
#16450=ORIENTED_EDGE('',*,*,#12404,.T.);
#16451=ORIENTED_EDGE('',*,*,#12403,.F.);
#16452=ORIENTED_EDGE('',*,*,#12405,.T.);
#16453=ORIENTED_EDGE('',*,*,#12406,.T.);
#16454=ORIENTED_EDGE('',*,*,#12407,.T.);
#16455=ORIENTED_EDGE('',*,*,#12408,.F.);
#16456=ORIENTED_EDGE('',*,*,#12409,.T.);
#16457=ORIENTED_EDGE('',*,*,#12401,.T.);
#16458=ORIENTED_EDGE('',*,*,#12410,.T.);
#16459=ORIENTED_EDGE('',*,*,#12411,.F.);
#16460=ORIENTED_EDGE('',*,*,#12412,.T.);
#16461=ORIENTED_EDGE('',*,*,#12408,.T.);
#16462=ORIENTED_EDGE('',*,*,#12413,.T.);
#16463=ORIENTED_EDGE('',*,*,#12414,.F.);
#16464=ORIENTED_EDGE('',*,*,#12415,.T.);
#16465=ORIENTED_EDGE('',*,*,#12411,.T.);
#16466=ORIENTED_EDGE('',*,*,#12416,.T.);
#16467=ORIENTED_EDGE('',*,*,#12417,.F.);
#16468=ORIENTED_EDGE('',*,*,#12418,.T.);
#16469=ORIENTED_EDGE('',*,*,#12414,.T.);
#16470=ORIENTED_EDGE('',*,*,#12419,.T.);
#16471=ORIENTED_EDGE('',*,*,#12420,.F.);
#16472=ORIENTED_EDGE('',*,*,#12421,.T.);
#16473=ORIENTED_EDGE('',*,*,#12417,.T.);
#16474=ORIENTED_EDGE('',*,*,#12422,.T.);
#16475=ORIENTED_EDGE('',*,*,#12423,.F.);
#16476=ORIENTED_EDGE('',*,*,#12424,.T.);
#16477=ORIENTED_EDGE('',*,*,#12420,.T.);
#16478=ORIENTED_EDGE('',*,*,#12425,.T.);
#16479=ORIENTED_EDGE('',*,*,#12426,.F.);
#16480=ORIENTED_EDGE('',*,*,#12427,.T.);
#16481=ORIENTED_EDGE('',*,*,#12423,.T.);
#16482=ORIENTED_EDGE('',*,*,#12428,.T.);
#16483=ORIENTED_EDGE('',*,*,#12429,.F.);
#16484=ORIENTED_EDGE('',*,*,#12430,.T.);
#16485=ORIENTED_EDGE('',*,*,#12426,.T.);
#16486=ORIENTED_EDGE('',*,*,#12431,.T.);
#16487=ORIENTED_EDGE('',*,*,#12432,.F.);
#16488=ORIENTED_EDGE('',*,*,#12433,.T.);
#16489=ORIENTED_EDGE('',*,*,#12429,.T.);
#16490=ORIENTED_EDGE('',*,*,#12434,.T.);
#16491=ORIENTED_EDGE('',*,*,#12435,.F.);
#16492=ORIENTED_EDGE('',*,*,#12436,.T.);
#16493=ORIENTED_EDGE('',*,*,#12437,.F.);
#16494=ORIENTED_EDGE('',*,*,#12438,.F.);
#16495=ORIENTED_EDGE('',*,*,#12439,.F.);
#16496=ORIENTED_EDGE('',*,*,#12440,.T.);
#16497=ORIENTED_EDGE('',*,*,#12435,.T.);
#16498=ORIENTED_EDGE('',*,*,#12441,.F.);
#16499=ORIENTED_EDGE('',*,*,#12442,.F.);
#16500=ORIENTED_EDGE('',*,*,#12443,.T.);
#16501=ORIENTED_EDGE('',*,*,#12439,.T.);
#16502=ORIENTED_EDGE('',*,*,#12444,.F.);
#16503=ORIENTED_EDGE('',*,*,#12445,.F.);
#16504=ORIENTED_EDGE('',*,*,#12446,.T.);
#16505=ORIENTED_EDGE('',*,*,#12442,.T.);
#16506=ORIENTED_EDGE('',*,*,#12447,.F.);
#16507=ORIENTED_EDGE('',*,*,#12448,.F.);
#16508=ORIENTED_EDGE('',*,*,#12449,.T.);
#16509=ORIENTED_EDGE('',*,*,#12445,.T.);
#16510=ORIENTED_EDGE('',*,*,#12450,.F.);
#16511=ORIENTED_EDGE('',*,*,#12451,.F.);
#16512=ORIENTED_EDGE('',*,*,#12452,.T.);
#16513=ORIENTED_EDGE('',*,*,#12448,.T.);
#16514=ORIENTED_EDGE('',*,*,#12453,.F.);
#16515=ORIENTED_EDGE('',*,*,#12454,.F.);
#16516=ORIENTED_EDGE('',*,*,#12455,.T.);
#16517=ORIENTED_EDGE('',*,*,#12451,.T.);
#16518=ORIENTED_EDGE('',*,*,#12456,.F.);
#16519=ORIENTED_EDGE('',*,*,#12457,.F.);
#16520=ORIENTED_EDGE('',*,*,#12458,.T.);
#16521=ORIENTED_EDGE('',*,*,#12454,.T.);
#16522=ORIENTED_EDGE('',*,*,#12459,.F.);
#16523=ORIENTED_EDGE('',*,*,#12460,.F.);
#16524=ORIENTED_EDGE('',*,*,#12461,.T.);
#16525=ORIENTED_EDGE('',*,*,#12457,.T.);
#16526=ORIENTED_EDGE('',*,*,#12462,.F.);
#16527=ORIENTED_EDGE('',*,*,#12463,.F.);
#16528=ORIENTED_EDGE('',*,*,#12464,.T.);
#16529=ORIENTED_EDGE('',*,*,#12460,.T.);
#16530=ORIENTED_EDGE('',*,*,#12465,.F.);
#16531=ORIENTED_EDGE('',*,*,#12466,.F.);
#16532=ORIENTED_EDGE('',*,*,#12467,.T.);
#16533=ORIENTED_EDGE('',*,*,#12463,.T.);
#16534=ORIENTED_EDGE('',*,*,#12468,.F.);
#16535=ORIENTED_EDGE('',*,*,#12469,.F.);
#16536=ORIENTED_EDGE('',*,*,#12470,.F.);
#16537=ORIENTED_EDGE('',*,*,#12434,.F.);
#16538=ORIENTED_EDGE('',*,*,#12431,.F.);
#16539=ORIENTED_EDGE('',*,*,#12428,.F.);
#16540=ORIENTED_EDGE('',*,*,#12425,.F.);
#16541=ORIENTED_EDGE('',*,*,#12422,.F.);
#16542=ORIENTED_EDGE('',*,*,#12419,.F.);
#16543=ORIENTED_EDGE('',*,*,#12416,.F.);
#16544=ORIENTED_EDGE('',*,*,#12413,.F.);
#16545=ORIENTED_EDGE('',*,*,#12410,.F.);
#16546=ORIENTED_EDGE('',*,*,#12407,.F.);
#16547=ORIENTED_EDGE('',*,*,#12471,.F.);
#16548=ORIENTED_EDGE('',*,*,#12472,.T.);
#16549=ORIENTED_EDGE('',*,*,#12468,.T.);
#16550=ORIENTED_EDGE('',*,*,#12465,.T.);
#16551=ORIENTED_EDGE('',*,*,#12462,.T.);
#16552=ORIENTED_EDGE('',*,*,#12459,.T.);
#16553=ORIENTED_EDGE('',*,*,#12456,.T.);
#16554=ORIENTED_EDGE('',*,*,#12453,.T.);
#16555=ORIENTED_EDGE('',*,*,#12450,.T.);
#16556=ORIENTED_EDGE('',*,*,#12447,.T.);
#16557=ORIENTED_EDGE('',*,*,#12444,.T.);
#16558=ORIENTED_EDGE('',*,*,#12441,.T.);
#16559=ORIENTED_EDGE('',*,*,#12438,.T.);
#16560=ORIENTED_EDGE('',*,*,#12406,.F.);
#16561=ORIENTED_EDGE('',*,*,#12473,.T.);
#16562=ORIENTED_EDGE('',*,*,#12474,.T.);
#16563=ORIENTED_EDGE('',*,*,#12471,.T.);
#16564=ORIENTED_EDGE('',*,*,#12466,.T.);
#16565=ORIENTED_EDGE('',*,*,#12472,.F.);
#16566=ORIENTED_EDGE('',*,*,#12474,.F.);
#16567=ORIENTED_EDGE('',*,*,#12475,.T.);
#16568=ORIENTED_EDGE('',*,*,#12476,.F.);
#16569=ORIENTED_EDGE('',*,*,#12436,.F.);
#16570=ORIENTED_EDGE('',*,*,#12440,.F.);
#16571=ORIENTED_EDGE('',*,*,#12443,.F.);
#16572=ORIENTED_EDGE('',*,*,#12446,.F.);
#16573=ORIENTED_EDGE('',*,*,#12449,.F.);
#16574=ORIENTED_EDGE('',*,*,#12452,.F.);
#16575=ORIENTED_EDGE('',*,*,#12455,.F.);
#16576=ORIENTED_EDGE('',*,*,#12458,.F.);
#16577=ORIENTED_EDGE('',*,*,#12461,.F.);
#16578=ORIENTED_EDGE('',*,*,#12464,.F.);
#16579=ORIENTED_EDGE('',*,*,#12467,.F.);
#16580=ORIENTED_EDGE('',*,*,#12475,.F.);
#16581=ORIENTED_EDGE('',*,*,#12473,.F.);
#16582=ORIENTED_EDGE('',*,*,#12405,.F.);
#16583=ORIENTED_EDGE('',*,*,#12402,.F.);
#16584=ORIENTED_EDGE('',*,*,#12409,.F.);
#16585=ORIENTED_EDGE('',*,*,#12412,.F.);
#16586=ORIENTED_EDGE('',*,*,#12415,.F.);
#16587=ORIENTED_EDGE('',*,*,#12418,.F.);
#16588=ORIENTED_EDGE('',*,*,#12421,.F.);
#16589=ORIENTED_EDGE('',*,*,#12424,.F.);
#16590=ORIENTED_EDGE('',*,*,#12427,.F.);
#16591=ORIENTED_EDGE('',*,*,#12430,.F.);
#16592=ORIENTED_EDGE('',*,*,#12433,.F.);
#16593=ORIENTED_EDGE('',*,*,#12477,.F.);
#16594=ORIENTED_EDGE('',*,*,#12478,.F.);
#16595=ORIENTED_EDGE('',*,*,#12479,.T.);
#16596=ORIENTED_EDGE('',*,*,#12480,.F.);
#16597=ORIENTED_EDGE('',*,*,#12479,.F.);
#16598=ORIENTED_EDGE('',*,*,#12481,.F.);
#16599=ORIENTED_EDGE('',*,*,#12482,.T.);
#16600=ORIENTED_EDGE('',*,*,#12483,.F.);
#16601=ORIENTED_EDGE('',*,*,#12482,.F.);
#16602=ORIENTED_EDGE('',*,*,#12484,.F.);
#16603=ORIENTED_EDGE('',*,*,#12485,.T.);
#16604=ORIENTED_EDGE('',*,*,#12486,.F.);
#16605=ORIENTED_EDGE('',*,*,#12485,.F.);
#16606=ORIENTED_EDGE('',*,*,#12487,.F.);
#16607=ORIENTED_EDGE('',*,*,#12488,.T.);
#16608=ORIENTED_EDGE('',*,*,#12489,.F.);
#16609=ORIENTED_EDGE('',*,*,#12488,.F.);
#16610=ORIENTED_EDGE('',*,*,#12490,.F.);
#16611=ORIENTED_EDGE('',*,*,#12491,.F.);
#16612=ORIENTED_EDGE('',*,*,#12492,.T.);
#16613=ORIENTED_EDGE('',*,*,#12493,.T.);
#16614=ORIENTED_EDGE('',*,*,#12494,.F.);
#16615=ORIENTED_EDGE('',*,*,#12493,.F.);
#16616=ORIENTED_EDGE('',*,*,#12495,.F.);
#16617=ORIENTED_EDGE('',*,*,#12496,.F.);
#16618=ORIENTED_EDGE('',*,*,#12495,.T.);
#16619=ORIENTED_EDGE('',*,*,#12492,.F.);
#16620=ORIENTED_EDGE('',*,*,#12497,.F.);
#16621=ORIENTED_EDGE('',*,*,#12498,.F.);
#16622=ORIENTED_EDGE('',*,*,#12497,.T.);
#16623=ORIENTED_EDGE('',*,*,#12491,.T.);
#16624=ORIENTED_EDGE('',*,*,#12499,.F.);
#16625=ORIENTED_EDGE('',*,*,#12500,.F.);
#16626=ORIENTED_EDGE('',*,*,#12501,.T.);
#16627=ORIENTED_EDGE('',*,*,#12502,.T.);
#16628=ORIENTED_EDGE('',*,*,#12503,.F.);
#16629=ORIENTED_EDGE('',*,*,#12502,.F.);
#16630=ORIENTED_EDGE('',*,*,#12504,.F.);
#16631=ORIENTED_EDGE('',*,*,#12505,.F.);
#16632=ORIENTED_EDGE('',*,*,#12504,.T.);
#16633=ORIENTED_EDGE('',*,*,#12501,.F.);
#16634=ORIENTED_EDGE('',*,*,#12506,.F.);
#16635=ORIENTED_EDGE('',*,*,#12507,.F.);
#16636=ORIENTED_EDGE('',*,*,#12506,.T.);
#16637=ORIENTED_EDGE('',*,*,#12500,.T.);
#16638=ORIENTED_EDGE('',*,*,#12508,.F.);
#16639=ORIENTED_EDGE('',*,*,#12509,.F.);
#16640=ORIENTED_EDGE('',*,*,#12510,.T.);
#16641=ORIENTED_EDGE('',*,*,#12511,.T.);
#16642=ORIENTED_EDGE('',*,*,#12512,.F.);
#16643=ORIENTED_EDGE('',*,*,#12511,.F.);
#16644=ORIENTED_EDGE('',*,*,#12513,.F.);
#16645=ORIENTED_EDGE('',*,*,#12514,.F.);
#16646=ORIENTED_EDGE('',*,*,#12513,.T.);
#16647=ORIENTED_EDGE('',*,*,#12510,.F.);
#16648=ORIENTED_EDGE('',*,*,#12515,.F.);
#16649=ORIENTED_EDGE('',*,*,#12516,.F.);
#16650=ORIENTED_EDGE('',*,*,#12515,.T.);
#16651=ORIENTED_EDGE('',*,*,#12509,.T.);
#16652=ORIENTED_EDGE('',*,*,#12517,.F.);
#16653=ORIENTED_EDGE('',*,*,#12518,.F.);
#16654=ORIENTED_EDGE('',*,*,#12519,.T.);
#16655=ORIENTED_EDGE('',*,*,#12520,.T.);
#16656=ORIENTED_EDGE('',*,*,#12521,.F.);
#16657=ORIENTED_EDGE('',*,*,#12520,.F.);
#16658=ORIENTED_EDGE('',*,*,#12522,.F.);
#16659=ORIENTED_EDGE('',*,*,#12523,.F.);
#16660=ORIENTED_EDGE('',*,*,#12522,.T.);
#16661=ORIENTED_EDGE('',*,*,#12519,.F.);
#16662=ORIENTED_EDGE('',*,*,#12524,.F.);
#16663=ORIENTED_EDGE('',*,*,#12525,.F.);
#16664=ORIENTED_EDGE('',*,*,#12524,.T.);
#16665=ORIENTED_EDGE('',*,*,#12518,.T.);
#16666=ORIENTED_EDGE('',*,*,#12526,.F.);
#16667=ORIENTED_EDGE('',*,*,#12527,.F.);
#16668=ORIENTED_EDGE('',*,*,#12528,.T.);
#16669=ORIENTED_EDGE('',*,*,#12529,.T.);
#16670=ORIENTED_EDGE('',*,*,#12530,.F.);
#16671=ORIENTED_EDGE('',*,*,#12529,.F.);
#16672=ORIENTED_EDGE('',*,*,#12531,.F.);
#16673=ORIENTED_EDGE('',*,*,#12532,.F.);
#16674=ORIENTED_EDGE('',*,*,#12531,.T.);
#16675=ORIENTED_EDGE('',*,*,#12528,.F.);
#16676=ORIENTED_EDGE('',*,*,#12533,.F.);
#16677=ORIENTED_EDGE('',*,*,#12534,.F.);
#16678=ORIENTED_EDGE('',*,*,#12533,.T.);
#16679=ORIENTED_EDGE('',*,*,#12527,.T.);
#16680=ORIENTED_EDGE('',*,*,#12535,.F.);
#16681=ORIENTED_EDGE('',*,*,#12536,.F.);
#16682=ORIENTED_EDGE('',*,*,#12537,.T.);
#16683=ORIENTED_EDGE('',*,*,#12538,.T.);
#16684=ORIENTED_EDGE('',*,*,#12539,.F.);
#16685=ORIENTED_EDGE('',*,*,#12538,.F.);
#16686=ORIENTED_EDGE('',*,*,#12540,.F.);
#16687=ORIENTED_EDGE('',*,*,#12541,.F.);
#16688=ORIENTED_EDGE('',*,*,#12540,.T.);
#16689=ORIENTED_EDGE('',*,*,#12537,.F.);
#16690=ORIENTED_EDGE('',*,*,#12542,.F.);
#16691=ORIENTED_EDGE('',*,*,#12543,.F.);
#16692=ORIENTED_EDGE('',*,*,#12542,.T.);
#16693=ORIENTED_EDGE('',*,*,#12536,.T.);
#16694=ORIENTED_EDGE('',*,*,#12544,.F.);
#16695=ORIENTED_EDGE('',*,*,#12545,.F.);
#16696=ORIENTED_EDGE('',*,*,#12546,.T.);
#16697=ORIENTED_EDGE('',*,*,#12547,.T.);
#16698=ORIENTED_EDGE('',*,*,#12548,.F.);
#16699=ORIENTED_EDGE('',*,*,#12547,.F.);
#16700=ORIENTED_EDGE('',*,*,#12549,.F.);
#16701=ORIENTED_EDGE('',*,*,#12550,.F.);
#16702=ORIENTED_EDGE('',*,*,#12549,.T.);
#16703=ORIENTED_EDGE('',*,*,#12546,.F.);
#16704=ORIENTED_EDGE('',*,*,#12551,.F.);
#16705=ORIENTED_EDGE('',*,*,#12552,.F.);
#16706=ORIENTED_EDGE('',*,*,#12551,.T.);
#16707=ORIENTED_EDGE('',*,*,#12545,.T.);
#16708=ORIENTED_EDGE('',*,*,#12553,.F.);
#16709=ORIENTED_EDGE('',*,*,#12554,.F.);
#16710=ORIENTED_EDGE('',*,*,#12555,.T.);
#16711=ORIENTED_EDGE('',*,*,#12556,.T.);
#16712=ORIENTED_EDGE('',*,*,#12557,.F.);
#16713=ORIENTED_EDGE('',*,*,#12556,.F.);
#16714=ORIENTED_EDGE('',*,*,#12558,.F.);
#16715=ORIENTED_EDGE('',*,*,#12559,.F.);
#16716=ORIENTED_EDGE('',*,*,#12558,.T.);
#16717=ORIENTED_EDGE('',*,*,#12555,.F.);
#16718=ORIENTED_EDGE('',*,*,#12560,.F.);
#16719=ORIENTED_EDGE('',*,*,#12561,.F.);
#16720=ORIENTED_EDGE('',*,*,#12560,.T.);
#16721=ORIENTED_EDGE('',*,*,#12554,.T.);
#16722=ORIENTED_EDGE('',*,*,#12562,.F.);
#16723=ORIENTED_EDGE('',*,*,#12563,.F.);
#16724=ORIENTED_EDGE('',*,*,#12564,.T.);
#16725=ORIENTED_EDGE('',*,*,#12565,.T.);
#16726=ORIENTED_EDGE('',*,*,#12566,.F.);
#16727=ORIENTED_EDGE('',*,*,#12565,.F.);
#16728=ORIENTED_EDGE('',*,*,#12567,.F.);
#16729=ORIENTED_EDGE('',*,*,#12568,.F.);
#16730=ORIENTED_EDGE('',*,*,#12567,.T.);
#16731=ORIENTED_EDGE('',*,*,#12564,.F.);
#16732=ORIENTED_EDGE('',*,*,#12569,.F.);
#16733=ORIENTED_EDGE('',*,*,#12570,.F.);
#16734=ORIENTED_EDGE('',*,*,#12569,.T.);
#16735=ORIENTED_EDGE('',*,*,#12563,.T.);
#16736=ORIENTED_EDGE('',*,*,#12571,.F.);
#16737=ORIENTED_EDGE('',*,*,#12572,.F.);
#16738=ORIENTED_EDGE('',*,*,#12573,.T.);
#16739=ORIENTED_EDGE('',*,*,#12574,.T.);
#16740=ORIENTED_EDGE('',*,*,#12575,.F.);
#16741=ORIENTED_EDGE('',*,*,#12574,.F.);
#16742=ORIENTED_EDGE('',*,*,#12576,.F.);
#16743=ORIENTED_EDGE('',*,*,#12577,.F.);
#16744=ORIENTED_EDGE('',*,*,#12576,.T.);
#16745=ORIENTED_EDGE('',*,*,#12573,.F.);
#16746=ORIENTED_EDGE('',*,*,#12578,.F.);
#16747=ORIENTED_EDGE('',*,*,#12579,.F.);
#16748=ORIENTED_EDGE('',*,*,#12578,.T.);
#16749=ORIENTED_EDGE('',*,*,#12572,.T.);
#16750=ORIENTED_EDGE('',*,*,#12580,.F.);
#16751=ORIENTED_EDGE('',*,*,#12581,.F.);
#16752=ORIENTED_EDGE('',*,*,#12582,.T.);
#16753=ORIENTED_EDGE('',*,*,#12583,.T.);
#16754=ORIENTED_EDGE('',*,*,#12584,.F.);
#16755=ORIENTED_EDGE('',*,*,#12583,.F.);
#16756=ORIENTED_EDGE('',*,*,#12585,.F.);
#16757=ORIENTED_EDGE('',*,*,#12586,.F.);
#16758=ORIENTED_EDGE('',*,*,#12585,.T.);
#16759=ORIENTED_EDGE('',*,*,#12582,.F.);
#16760=ORIENTED_EDGE('',*,*,#12587,.F.);
#16761=ORIENTED_EDGE('',*,*,#12588,.F.);
#16762=ORIENTED_EDGE('',*,*,#12587,.T.);
#16763=ORIENTED_EDGE('',*,*,#12581,.T.);
#16764=ORIENTED_EDGE('',*,*,#12589,.F.);
#16765=ORIENTED_EDGE('',*,*,#12590,.F.);
#16766=ORIENTED_EDGE('',*,*,#12591,.T.);
#16767=ORIENTED_EDGE('',*,*,#12592,.T.);
#16768=ORIENTED_EDGE('',*,*,#12593,.F.);
#16769=ORIENTED_EDGE('',*,*,#12592,.F.);
#16770=ORIENTED_EDGE('',*,*,#12594,.F.);
#16771=ORIENTED_EDGE('',*,*,#12595,.F.);
#16772=ORIENTED_EDGE('',*,*,#12596,.F.);
#16773=ORIENTED_EDGE('',*,*,#12594,.T.);
#16774=ORIENTED_EDGE('',*,*,#12591,.F.);
#16775=ORIENTED_EDGE('',*,*,#12597,.F.);
#16776=ORIENTED_EDGE('',*,*,#12598,.F.);
#16777=ORIENTED_EDGE('',*,*,#12597,.T.);
#16778=ORIENTED_EDGE('',*,*,#12590,.T.);
#16779=ORIENTED_EDGE('',*,*,#12599,.F.);
#16780=ORIENTED_EDGE('',*,*,#12600,.F.);
#16781=ORIENTED_EDGE('',*,*,#12601,.F.);
#16782=ORIENTED_EDGE('',*,*,#12602,.T.);
#16783=ORIENTED_EDGE('',*,*,#12603,.T.);
#16784=ORIENTED_EDGE('',*,*,#12604,.F.);
#16785=ORIENTED_EDGE('',*,*,#12603,.F.);
#16786=ORIENTED_EDGE('',*,*,#12605,.F.);
#16787=ORIENTED_EDGE('',*,*,#12606,.F.);
#16788=ORIENTED_EDGE('',*,*,#12605,.T.);
#16789=ORIENTED_EDGE('',*,*,#12602,.F.);
#16790=ORIENTED_EDGE('',*,*,#12607,.F.);
#16791=ORIENTED_EDGE('',*,*,#12608,.F.);
#16792=ORIENTED_EDGE('',*,*,#12607,.T.);
#16793=ORIENTED_EDGE('',*,*,#12601,.T.);
#16794=ORIENTED_EDGE('',*,*,#12609,.F.);
#16795=ORIENTED_EDGE('',*,*,#12610,.F.);
#16796=ORIENTED_EDGE('',*,*,#12611,.T.);
#16797=ORIENTED_EDGE('',*,*,#12612,.T.);
#16798=ORIENTED_EDGE('',*,*,#12613,.F.);
#16799=ORIENTED_EDGE('',*,*,#12612,.F.);
#16800=ORIENTED_EDGE('',*,*,#12614,.F.);
#16801=ORIENTED_EDGE('',*,*,#12615,.F.);
#16802=ORIENTED_EDGE('',*,*,#12614,.T.);
#16803=ORIENTED_EDGE('',*,*,#12611,.F.);
#16804=ORIENTED_EDGE('',*,*,#12616,.F.);
#16805=ORIENTED_EDGE('',*,*,#12617,.F.);
#16806=ORIENTED_EDGE('',*,*,#12616,.T.);
#16807=ORIENTED_EDGE('',*,*,#12610,.T.);
#16808=ORIENTED_EDGE('',*,*,#12618,.F.);
#16809=ORIENTED_EDGE('',*,*,#12619,.F.);
#16810=ORIENTED_EDGE('',*,*,#12620,.T.);
#16811=ORIENTED_EDGE('',*,*,#12621,.T.);
#16812=ORIENTED_EDGE('',*,*,#12622,.F.);
#16813=ORIENTED_EDGE('',*,*,#12621,.F.);
#16814=ORIENTED_EDGE('',*,*,#12623,.F.);
#16815=ORIENTED_EDGE('',*,*,#12624,.F.);
#16816=ORIENTED_EDGE('',*,*,#12623,.T.);
#16817=ORIENTED_EDGE('',*,*,#12620,.F.);
#16818=ORIENTED_EDGE('',*,*,#12625,.F.);
#16819=ORIENTED_EDGE('',*,*,#12626,.F.);
#16820=ORIENTED_EDGE('',*,*,#12625,.T.);
#16821=ORIENTED_EDGE('',*,*,#12619,.T.);
#16822=ORIENTED_EDGE('',*,*,#12627,.F.);
#16823=ORIENTED_EDGE('',*,*,#12628,.F.);
#16824=ORIENTED_EDGE('',*,*,#12629,.T.);
#16825=ORIENTED_EDGE('',*,*,#12630,.T.);
#16826=ORIENTED_EDGE('',*,*,#12631,.F.);
#16827=ORIENTED_EDGE('',*,*,#12630,.F.);
#16828=ORIENTED_EDGE('',*,*,#12632,.F.);
#16829=ORIENTED_EDGE('',*,*,#12633,.F.);
#16830=ORIENTED_EDGE('',*,*,#12632,.T.);
#16831=ORIENTED_EDGE('',*,*,#12629,.F.);
#16832=ORIENTED_EDGE('',*,*,#12634,.F.);
#16833=ORIENTED_EDGE('',*,*,#12635,.F.);
#16834=ORIENTED_EDGE('',*,*,#12634,.T.);
#16835=ORIENTED_EDGE('',*,*,#12628,.T.);
#16836=ORIENTED_EDGE('',*,*,#12636,.F.);
#16837=ORIENTED_EDGE('',*,*,#12637,.F.);
#16838=ORIENTED_EDGE('',*,*,#12638,.T.);
#16839=ORIENTED_EDGE('',*,*,#12639,.T.);
#16840=ORIENTED_EDGE('',*,*,#12640,.F.);
#16841=ORIENTED_EDGE('',*,*,#12639,.F.);
#16842=ORIENTED_EDGE('',*,*,#12641,.F.);
#16843=ORIENTED_EDGE('',*,*,#12642,.F.);
#16844=ORIENTED_EDGE('',*,*,#12641,.T.);
#16845=ORIENTED_EDGE('',*,*,#12638,.F.);
#16846=ORIENTED_EDGE('',*,*,#12643,.F.);
#16847=ORIENTED_EDGE('',*,*,#12644,.F.);
#16848=ORIENTED_EDGE('',*,*,#12643,.T.);
#16849=ORIENTED_EDGE('',*,*,#12637,.T.);
#16850=ORIENTED_EDGE('',*,*,#12645,.F.);
#16851=ORIENTED_EDGE('',*,*,#12646,.F.);
#16852=ORIENTED_EDGE('',*,*,#12647,.T.);
#16853=ORIENTED_EDGE('',*,*,#12648,.T.);
#16854=ORIENTED_EDGE('',*,*,#12649,.F.);
#16855=ORIENTED_EDGE('',*,*,#12648,.F.);
#16856=ORIENTED_EDGE('',*,*,#12650,.F.);
#16857=ORIENTED_EDGE('',*,*,#12651,.F.);
#16858=ORIENTED_EDGE('',*,*,#12650,.T.);
#16859=ORIENTED_EDGE('',*,*,#12647,.F.);
#16860=ORIENTED_EDGE('',*,*,#12652,.F.);
#16861=ORIENTED_EDGE('',*,*,#12653,.F.);
#16862=ORIENTED_EDGE('',*,*,#12652,.T.);
#16863=ORIENTED_EDGE('',*,*,#12646,.T.);
#16864=ORIENTED_EDGE('',*,*,#12654,.F.);
#16865=ORIENTED_EDGE('',*,*,#12655,.F.);
#16866=ORIENTED_EDGE('',*,*,#12656,.T.);
#16867=ORIENTED_EDGE('',*,*,#12657,.T.);
#16868=ORIENTED_EDGE('',*,*,#12658,.F.);
#16869=ORIENTED_EDGE('',*,*,#12657,.F.);
#16870=ORIENTED_EDGE('',*,*,#12659,.F.);
#16871=ORIENTED_EDGE('',*,*,#12660,.F.);
#16872=ORIENTED_EDGE('',*,*,#12659,.T.);
#16873=ORIENTED_EDGE('',*,*,#12656,.F.);
#16874=ORIENTED_EDGE('',*,*,#12661,.F.);
#16875=ORIENTED_EDGE('',*,*,#12662,.F.);
#16876=ORIENTED_EDGE('',*,*,#12661,.T.);
#16877=ORIENTED_EDGE('',*,*,#12655,.T.);
#16878=ORIENTED_EDGE('',*,*,#12663,.F.);
#16879=ORIENTED_EDGE('',*,*,#12664,.F.);
#16880=ORIENTED_EDGE('',*,*,#12665,.T.);
#16881=ORIENTED_EDGE('',*,*,#12666,.T.);
#16882=ORIENTED_EDGE('',*,*,#12667,.F.);
#16883=ORIENTED_EDGE('',*,*,#12666,.F.);
#16884=ORIENTED_EDGE('',*,*,#12668,.F.);
#16885=ORIENTED_EDGE('',*,*,#12669,.F.);
#16886=ORIENTED_EDGE('',*,*,#12668,.T.);
#16887=ORIENTED_EDGE('',*,*,#12665,.F.);
#16888=ORIENTED_EDGE('',*,*,#12670,.F.);
#16889=ORIENTED_EDGE('',*,*,#12671,.F.);
#16890=ORIENTED_EDGE('',*,*,#12670,.T.);
#16891=ORIENTED_EDGE('',*,*,#12664,.T.);
#16892=ORIENTED_EDGE('',*,*,#12672,.F.);
#16893=ORIENTED_EDGE('',*,*,#12673,.F.);
#16894=ORIENTED_EDGE('',*,*,#12674,.T.);
#16895=ORIENTED_EDGE('',*,*,#12675,.T.);
#16896=ORIENTED_EDGE('',*,*,#12676,.F.);
#16897=ORIENTED_EDGE('',*,*,#12675,.F.);
#16898=ORIENTED_EDGE('',*,*,#12677,.F.);
#16899=ORIENTED_EDGE('',*,*,#12678,.F.);
#16900=ORIENTED_EDGE('',*,*,#12677,.T.);
#16901=ORIENTED_EDGE('',*,*,#12674,.F.);
#16902=ORIENTED_EDGE('',*,*,#12679,.F.);
#16903=ORIENTED_EDGE('',*,*,#12680,.F.);
#16904=ORIENTED_EDGE('',*,*,#12679,.T.);
#16905=ORIENTED_EDGE('',*,*,#12673,.T.);
#16906=ORIENTED_EDGE('',*,*,#12681,.F.);
#16907=ORIENTED_EDGE('',*,*,#12682,.F.);
#16908=ORIENTED_EDGE('',*,*,#12683,.T.);
#16909=ORIENTED_EDGE('',*,*,#12684,.T.);
#16910=ORIENTED_EDGE('',*,*,#12685,.F.);
#16911=ORIENTED_EDGE('',*,*,#12684,.F.);
#16912=ORIENTED_EDGE('',*,*,#12686,.F.);
#16913=ORIENTED_EDGE('',*,*,#12687,.F.);
#16914=ORIENTED_EDGE('',*,*,#12686,.T.);
#16915=ORIENTED_EDGE('',*,*,#12683,.F.);
#16916=ORIENTED_EDGE('',*,*,#12688,.F.);
#16917=ORIENTED_EDGE('',*,*,#12689,.F.);
#16918=ORIENTED_EDGE('',*,*,#12688,.T.);
#16919=ORIENTED_EDGE('',*,*,#12682,.T.);
#16920=ORIENTED_EDGE('',*,*,#12690,.F.);
#16921=ORIENTED_EDGE('',*,*,#12691,.F.);
#16922=ORIENTED_EDGE('',*,*,#12692,.T.);
#16923=ORIENTED_EDGE('',*,*,#12693,.T.);
#16924=ORIENTED_EDGE('',*,*,#12694,.F.);
#16925=ORIENTED_EDGE('',*,*,#12693,.F.);
#16926=ORIENTED_EDGE('',*,*,#12695,.F.);
#16927=ORIENTED_EDGE('',*,*,#12696,.F.);
#16928=ORIENTED_EDGE('',*,*,#12695,.T.);
#16929=ORIENTED_EDGE('',*,*,#12692,.F.);
#16930=ORIENTED_EDGE('',*,*,#12697,.F.);
#16931=ORIENTED_EDGE('',*,*,#12698,.F.);
#16932=ORIENTED_EDGE('',*,*,#12697,.T.);
#16933=ORIENTED_EDGE('',*,*,#12691,.T.);
#16934=ORIENTED_EDGE('',*,*,#12699,.F.);
#16935=ORIENTED_EDGE('',*,*,#12700,.F.);
#16936=ORIENTED_EDGE('',*,*,#12701,.T.);
#16937=ORIENTED_EDGE('',*,*,#12702,.T.);
#16938=ORIENTED_EDGE('',*,*,#12703,.F.);
#16939=ORIENTED_EDGE('',*,*,#12702,.F.);
#16940=ORIENTED_EDGE('',*,*,#12704,.F.);
#16941=ORIENTED_EDGE('',*,*,#12705,.F.);
#16942=ORIENTED_EDGE('',*,*,#12704,.T.);
#16943=ORIENTED_EDGE('',*,*,#12701,.F.);
#16944=ORIENTED_EDGE('',*,*,#12706,.F.);
#16945=ORIENTED_EDGE('',*,*,#12707,.F.);
#16946=ORIENTED_EDGE('',*,*,#12706,.T.);
#16947=ORIENTED_EDGE('',*,*,#12700,.T.);
#16948=ORIENTED_EDGE('',*,*,#12708,.F.);
#16949=ORIENTED_EDGE('',*,*,#12709,.T.);
#16950=ORIENTED_EDGE('',*,*,#12710,.F.);
#16951=ORIENTED_EDGE('',*,*,#12709,.F.);
#16952=ORIENTED_EDGE('',*,*,#12711,.F.);
#16953=ORIENTED_EDGE('',*,*,#12712,.T.);
#16954=ORIENTED_EDGE('',*,*,#12708,.T.);
#16955=ORIENTED_EDGE('',*,*,#12712,.F.);
#16956=ORIENTED_EDGE('',*,*,#12711,.T.);
#16957=ORIENTED_EDGE('',*,*,#12713,.T.);
#16958=ORIENTED_EDGE('',*,*,#12710,.T.);
#16959=ORIENTED_EDGE('',*,*,#12713,.F.);
#16960=ORIENTED_EDGE('',*,*,#12714,.T.);
#16961=ORIENTED_EDGE('',*,*,#12715,.F.);
#16962=ORIENTED_EDGE('',*,*,#12714,.F.);
#16963=ORIENTED_EDGE('',*,*,#12716,.F.);
#16964=ORIENTED_EDGE('',*,*,#12717,.T.);
#16965=ORIENTED_EDGE('',*,*,#12595,.T.);
#16966=ORIENTED_EDGE('',*,*,#12596,.T.);
#16967=ORIENTED_EDGE('',*,*,#12598,.T.);
#16968=ORIENTED_EDGE('',*,*,#12718,.T.);
#16969=ORIENTED_EDGE('',*,*,#12719,.F.);
#16970=ORIENTED_EDGE('',*,*,#12718,.F.);
#16971=ORIENTED_EDGE('',*,*,#12599,.T.);
#16972=ORIENTED_EDGE('',*,*,#12589,.T.);
#16973=ORIENTED_EDGE('',*,*,#12593,.T.);
#16974=ORIENTED_EDGE('',*,*,#12717,.F.);
#16975=ORIENTED_EDGE('',*,*,#12496,.T.);
#16976=ORIENTED_EDGE('',*,*,#12498,.T.);
#16977=ORIENTED_EDGE('',*,*,#12490,.T.);
#16978=ORIENTED_EDGE('',*,*,#12494,.T.);
#16979=ORIENTED_EDGE('',*,*,#12505,.T.);
#16980=ORIENTED_EDGE('',*,*,#12507,.T.);
#16981=ORIENTED_EDGE('',*,*,#12499,.T.);
#16982=ORIENTED_EDGE('',*,*,#12503,.T.);
#16983=ORIENTED_EDGE('',*,*,#12514,.T.);
#16984=ORIENTED_EDGE('',*,*,#12516,.T.);
#16985=ORIENTED_EDGE('',*,*,#12508,.T.);
#16986=ORIENTED_EDGE('',*,*,#12512,.T.);
#16987=ORIENTED_EDGE('',*,*,#12523,.T.);
#16988=ORIENTED_EDGE('',*,*,#12525,.T.);
#16989=ORIENTED_EDGE('',*,*,#12517,.T.);
#16990=ORIENTED_EDGE('',*,*,#12521,.T.);
#16991=ORIENTED_EDGE('',*,*,#12532,.T.);
#16992=ORIENTED_EDGE('',*,*,#12534,.T.);
#16993=ORIENTED_EDGE('',*,*,#12526,.T.);
#16994=ORIENTED_EDGE('',*,*,#12530,.T.);
#16995=ORIENTED_EDGE('',*,*,#12541,.T.);
#16996=ORIENTED_EDGE('',*,*,#12543,.T.);
#16997=ORIENTED_EDGE('',*,*,#12535,.T.);
#16998=ORIENTED_EDGE('',*,*,#12539,.T.);
#16999=ORIENTED_EDGE('',*,*,#12550,.T.);
#17000=ORIENTED_EDGE('',*,*,#12552,.T.);
#17001=ORIENTED_EDGE('',*,*,#12544,.T.);
#17002=ORIENTED_EDGE('',*,*,#12548,.T.);
#17003=ORIENTED_EDGE('',*,*,#12559,.T.);
#17004=ORIENTED_EDGE('',*,*,#12561,.T.);
#17005=ORIENTED_EDGE('',*,*,#12553,.T.);
#17006=ORIENTED_EDGE('',*,*,#12557,.T.);
#17007=ORIENTED_EDGE('',*,*,#12568,.T.);
#17008=ORIENTED_EDGE('',*,*,#12570,.T.);
#17009=ORIENTED_EDGE('',*,*,#12562,.T.);
#17010=ORIENTED_EDGE('',*,*,#12566,.T.);
#17011=ORIENTED_EDGE('',*,*,#12577,.T.);
#17012=ORIENTED_EDGE('',*,*,#12579,.T.);
#17013=ORIENTED_EDGE('',*,*,#12571,.T.);
#17014=ORIENTED_EDGE('',*,*,#12575,.T.);
#17015=ORIENTED_EDGE('',*,*,#12586,.T.);
#17016=ORIENTED_EDGE('',*,*,#12588,.T.);
#17017=ORIENTED_EDGE('',*,*,#12580,.T.);
#17018=ORIENTED_EDGE('',*,*,#12584,.T.);
#17019=ORIENTED_EDGE('',*,*,#12606,.T.);
#17020=ORIENTED_EDGE('',*,*,#12608,.T.);
#17021=ORIENTED_EDGE('',*,*,#12600,.T.);
#17022=ORIENTED_EDGE('',*,*,#12604,.T.);
#17023=ORIENTED_EDGE('',*,*,#12615,.T.);
#17024=ORIENTED_EDGE('',*,*,#12617,.T.);
#17025=ORIENTED_EDGE('',*,*,#12609,.T.);
#17026=ORIENTED_EDGE('',*,*,#12613,.T.);
#17027=ORIENTED_EDGE('',*,*,#12624,.T.);
#17028=ORIENTED_EDGE('',*,*,#12626,.T.);
#17029=ORIENTED_EDGE('',*,*,#12618,.T.);
#17030=ORIENTED_EDGE('',*,*,#12622,.T.);
#17031=ORIENTED_EDGE('',*,*,#12633,.T.);
#17032=ORIENTED_EDGE('',*,*,#12635,.T.);
#17033=ORIENTED_EDGE('',*,*,#12627,.T.);
#17034=ORIENTED_EDGE('',*,*,#12631,.T.);
#17035=ORIENTED_EDGE('',*,*,#12642,.T.);
#17036=ORIENTED_EDGE('',*,*,#12644,.T.);
#17037=ORIENTED_EDGE('',*,*,#12636,.T.);
#17038=ORIENTED_EDGE('',*,*,#12640,.T.);
#17039=ORIENTED_EDGE('',*,*,#12651,.T.);
#17040=ORIENTED_EDGE('',*,*,#12653,.T.);
#17041=ORIENTED_EDGE('',*,*,#12645,.T.);
#17042=ORIENTED_EDGE('',*,*,#12649,.T.);
#17043=ORIENTED_EDGE('',*,*,#12660,.T.);
#17044=ORIENTED_EDGE('',*,*,#12662,.T.);
#17045=ORIENTED_EDGE('',*,*,#12654,.T.);
#17046=ORIENTED_EDGE('',*,*,#12658,.T.);
#17047=ORIENTED_EDGE('',*,*,#12669,.T.);
#17048=ORIENTED_EDGE('',*,*,#12671,.T.);
#17049=ORIENTED_EDGE('',*,*,#12663,.T.);
#17050=ORIENTED_EDGE('',*,*,#12667,.T.);
#17051=ORIENTED_EDGE('',*,*,#12678,.T.);
#17052=ORIENTED_EDGE('',*,*,#12680,.T.);
#17053=ORIENTED_EDGE('',*,*,#12672,.T.);
#17054=ORIENTED_EDGE('',*,*,#12676,.T.);
#17055=ORIENTED_EDGE('',*,*,#12687,.T.);
#17056=ORIENTED_EDGE('',*,*,#12689,.T.);
#17057=ORIENTED_EDGE('',*,*,#12681,.T.);
#17058=ORIENTED_EDGE('',*,*,#12685,.T.);
#17059=ORIENTED_EDGE('',*,*,#12696,.T.);
#17060=ORIENTED_EDGE('',*,*,#12698,.T.);
#17061=ORIENTED_EDGE('',*,*,#12690,.T.);
#17062=ORIENTED_EDGE('',*,*,#12694,.T.);
#17063=ORIENTED_EDGE('',*,*,#12705,.T.);
#17064=ORIENTED_EDGE('',*,*,#12707,.T.);
#17065=ORIENTED_EDGE('',*,*,#12699,.T.);
#17066=ORIENTED_EDGE('',*,*,#12703,.T.);
#17067=ORIENTED_EDGE('',*,*,#12720,.F.);
#17068=ORIENTED_EDGE('',*,*,#12716,.T.);
#17069=ORIENTED_EDGE('',*,*,#12721,.F.);
#17070=ORIENTED_EDGE('',*,*,#12722,.T.);
#17071=ORIENTED_EDGE('',*,*,#12720,.T.);
#17072=ORIENTED_EDGE('',*,*,#12722,.F.);
#17073=ORIENTED_EDGE('',*,*,#12723,.F.);
#17074=ORIENTED_EDGE('',*,*,#12724,.T.);
#17075=ORIENTED_EDGE('',*,*,#12721,.T.);
#17076=ORIENTED_EDGE('',*,*,#12724,.F.);
#17077=ORIENTED_EDGE('',*,*,#12723,.T.);
#17078=ORIENTED_EDGE('',*,*,#12715,.T.);
#17079=ORIENTED_EDGE('',*,*,#12725,.F.);
#17080=ORIENTED_EDGE('',*,*,#12726,.T.);
#17081=ORIENTED_EDGE('',*,*,#12727,.F.);
#17082=ORIENTED_EDGE('',*,*,#12728,.F.);
#17083=ORIENTED_EDGE('',*,*,#12729,.F.);
#17084=ORIENTED_EDGE('',*,*,#12728,.T.);
#17085=ORIENTED_EDGE('',*,*,#12730,.F.);
#17086=ORIENTED_EDGE('',*,*,#12731,.F.);
#17087=ORIENTED_EDGE('',*,*,#12732,.F.);
#17088=ORIENTED_EDGE('',*,*,#12731,.T.);
#17089=ORIENTED_EDGE('',*,*,#12733,.F.);
#17090=ORIENTED_EDGE('',*,*,#12734,.F.);
#17091=ORIENTED_EDGE('',*,*,#12735,.F.);
#17092=ORIENTED_EDGE('',*,*,#12734,.T.);
#17093=ORIENTED_EDGE('',*,*,#12736,.F.);
#17094=ORIENTED_EDGE('',*,*,#12737,.F.);
#17095=ORIENTED_EDGE('',*,*,#12738,.F.);
#17096=ORIENTED_EDGE('',*,*,#12737,.T.);
#17097=ORIENTED_EDGE('',*,*,#12739,.F.);
#17098=ORIENTED_EDGE('',*,*,#12740,.F.);
#17099=ORIENTED_EDGE('',*,*,#12741,.F.);
#17100=ORIENTED_EDGE('',*,*,#12740,.T.);
#17101=ORIENTED_EDGE('',*,*,#12742,.F.);
#17102=ORIENTED_EDGE('',*,*,#12726,.F.);
#17103=ORIENTED_EDGE('',*,*,#12742,.T.);
#17104=ORIENTED_EDGE('',*,*,#12739,.T.);
#17105=ORIENTED_EDGE('',*,*,#12736,.T.);
#17106=ORIENTED_EDGE('',*,*,#12733,.T.);
#17107=ORIENTED_EDGE('',*,*,#12730,.T.);
#17108=ORIENTED_EDGE('',*,*,#12727,.T.);
#17109=ORIENTED_EDGE('',*,*,#12719,.T.);
#17110=ORIENTED_EDGE('',*,*,#12743,.F.);
#17111=ORIENTED_EDGE('',*,*,#12744,.F.);
#17112=ORIENTED_EDGE('',*,*,#12745,.F.);
#17113=ORIENTED_EDGE('',*,*,#12746,.F.);
#17114=ORIENTED_EDGE('',*,*,#12478,.T.);
#17115=ORIENTED_EDGE('',*,*,#12481,.T.);
#17116=ORIENTED_EDGE('',*,*,#12484,.T.);
#17117=ORIENTED_EDGE('',*,*,#12487,.T.);
#17118=ORIENTED_EDGE('',*,*,#12747,.T.);
#17119=ORIENTED_EDGE('',*,*,#12469,.T.);
#17120=ORIENTED_EDGE('',*,*,#12437,.T.);
#17121=ORIENTED_EDGE('',*,*,#12476,.T.);
#17122=ORIENTED_EDGE('',*,*,#12744,.T.);
#17123=ORIENTED_EDGE('',*,*,#12748,.T.);
#17124=ORIENTED_EDGE('',*,*,#12749,.F.);
#17125=ORIENTED_EDGE('',*,*,#12750,.F.);
#17126=ORIENTED_EDGE('',*,*,#12745,.T.);
#17127=ORIENTED_EDGE('',*,*,#12750,.T.);
#17128=ORIENTED_EDGE('',*,*,#12751,.F.);
#17129=ORIENTED_EDGE('',*,*,#12752,.F.);
#17130=ORIENTED_EDGE('',*,*,#12746,.T.);
#17131=ORIENTED_EDGE('',*,*,#12752,.T.);
#17132=ORIENTED_EDGE('',*,*,#12753,.F.);
#17133=ORIENTED_EDGE('',*,*,#12754,.F.);
#17134=ORIENTED_EDGE('',*,*,#12743,.T.);
#17135=ORIENTED_EDGE('',*,*,#12754,.T.);
#17136=ORIENTED_EDGE('',*,*,#12755,.F.);
#17137=ORIENTED_EDGE('',*,*,#12748,.F.);
#17138=ORIENTED_EDGE('',*,*,#12755,.T.);
#17139=ORIENTED_EDGE('',*,*,#12753,.T.);
#17140=ORIENTED_EDGE('',*,*,#12751,.T.);
#17141=ORIENTED_EDGE('',*,*,#12749,.T.);
#17142=ORIENTED_EDGE('',*,*,#12480,.T.);
#17143=ORIENTED_EDGE('',*,*,#12483,.T.);
#17144=ORIENTED_EDGE('',*,*,#12486,.T.);
#17145=ORIENTED_EDGE('',*,*,#12489,.T.);
#17146=ORIENTED_EDGE('',*,*,#12725,.T.);
#17147=ORIENTED_EDGE('',*,*,#12729,.T.);
#17148=ORIENTED_EDGE('',*,*,#12732,.T.);
#17149=ORIENTED_EDGE('',*,*,#12735,.T.);
#17150=ORIENTED_EDGE('',*,*,#12738,.T.);
#17151=ORIENTED_EDGE('',*,*,#12741,.T.);
#17152=ORIENTED_EDGE('',*,*,#12756,.F.);
#17153=ORIENTED_EDGE('',*,*,#12404,.F.);
#17154=ORIENTED_EDGE('',*,*,#12757,.T.);
#17155=ORIENTED_EDGE('',*,*,#12756,.T.);
#17156=ORIENTED_EDGE('',*,*,#12757,.F.);
#17157=ORIENTED_EDGE('',*,*,#12432,.T.);
#17158=ORIENTED_EDGE('',*,*,#12470,.T.);
#17159=ORIENTED_EDGE('',*,*,#12747,.F.);
#17160=ORIENTED_EDGE('',*,*,#12477,.T.);
#21936=CONICAL_SURFACE('',#24296,0.045,0.643501108793287);
#21937=CONICAL_SURFACE('',#24310,0.5,0.785398163397451);
#21938=CONICAL_SURFACE('',#24329,0.38,0.785398163397448);
#22294=ADVANCED_FACE('',(#2555),#1000,.T.);
#22295=ADVANCED_FACE('',(#2556),#1001,.T.);
#22296=ADVANCED_FACE('',(#2557),#1002,.T.);
#22297=ADVANCED_FACE('',(#2558),#1003,.T.);
#22298=ADVANCED_FACE('',(#2559),#1004,.T.);
#22299=ADVANCED_FACE('',(#2560),#1005,.T.);
#22300=ADVANCED_FACE('',(#2561),#1006,.T.);
#22301=ADVANCED_FACE('',(#2562),#1007,.T.);
#22302=ADVANCED_FACE('',(#2563),#1008,.T.);
#22303=ADVANCED_FACE('',(#2564),#1009,.T.);
#22304=ADVANCED_FACE('',(#2565),#1010,.T.);
#22305=ADVANCED_FACE('',(#2566),#1011,.T.);
#22306=ADVANCED_FACE('',(#2567),#1012,.T.);
#22307=ADVANCED_FACE('',(#2568),#1013,.T.);
#22308=ADVANCED_FACE('',(#2569),#1014,.T.);
#22309=ADVANCED_FACE('',(#2570),#1015,.T.);
#22310=ADVANCED_FACE('',(#2571),#1016,.T.);
#22311=ADVANCED_FACE('',(#2572),#1017,.T.);
#22312=ADVANCED_FACE('',(#2573),#1018,.T.);
#22313=ADVANCED_FACE('',(#2574),#1019,.T.);
#22314=ADVANCED_FACE('',(#2575),#1020,.T.);
#22315=ADVANCED_FACE('',(#2576),#363,.F.);
#22316=ADVANCED_FACE('',(#2577),#1553,.T.);
#22317=ADVANCED_FACE('',(#2578),#1021,.T.);
#22318=ADVANCED_FACE('',(#2579),#364,.F.);
#22319=ADVANCED_FACE('',(#2580),#1022,.F.);
#22320=ADVANCED_FACE('',(#2581),#1023,.F.);
#22321=ADVANCED_FACE('',(#2582),#1024,.F.);
#22322=ADVANCED_FACE('',(#2583),#1025,.F.);
#22323=ADVANCED_FACE('',(#2584),#1554,.F.);
#22324=ADVANCED_FACE('',(#2585),#1555,.F.);
#22325=ADVANCED_FACE('',(#2586),#1556,.F.);
#22326=ADVANCED_FACE('',(#2587),#1557,.T.);
#22327=ADVANCED_FACE('',(#2588),#1558,.F.);
#22328=ADVANCED_FACE('',(#2589),#1559,.F.);
#22329=ADVANCED_FACE('',(#2590),#1560,.F.);
#22330=ADVANCED_FACE('',(#2591),#1561,.T.);
#22331=ADVANCED_FACE('',(#2592),#1562,.F.);
#22332=ADVANCED_FACE('',(#2593),#1563,.F.);
#22333=ADVANCED_FACE('',(#2594),#1564,.F.);
#22334=ADVANCED_FACE('',(#2595),#1565,.T.);
#22335=ADVANCED_FACE('',(#2596),#1566,.F.);
#22336=ADVANCED_FACE('',(#2597),#1567,.F.);
#22337=ADVANCED_FACE('',(#2598),#1568,.F.);
#22338=ADVANCED_FACE('',(#2599),#1569,.T.);
#22339=ADVANCED_FACE('',(#2600),#1570,.F.);
#22340=ADVANCED_FACE('',(#2601),#1571,.F.);
#22341=ADVANCED_FACE('',(#2602),#1572,.F.);
#22342=ADVANCED_FACE('',(#2603),#1573,.T.);
#22343=ADVANCED_FACE('',(#2604),#1574,.F.);
#22344=ADVANCED_FACE('',(#2605),#1575,.F.);
#22345=ADVANCED_FACE('',(#2606),#1576,.F.);
#22346=ADVANCED_FACE('',(#2607),#1577,.T.);
#22347=ADVANCED_FACE('',(#2608),#1578,.F.);
#22348=ADVANCED_FACE('',(#2609),#1579,.F.);
#22349=ADVANCED_FACE('',(#2610),#1580,.F.);
#22350=ADVANCED_FACE('',(#2611),#1581,.T.);
#22351=ADVANCED_FACE('',(#2612),#1582,.F.);
#22352=ADVANCED_FACE('',(#2613),#1583,.F.);
#22353=ADVANCED_FACE('',(#2614),#1584,.F.);
#22354=ADVANCED_FACE('',(#2615),#1585,.T.);
#22355=ADVANCED_FACE('',(#2616),#1586,.F.);
#22356=ADVANCED_FACE('',(#2617),#1587,.F.);
#22357=ADVANCED_FACE('',(#2618),#1588,.F.);
#22358=ADVANCED_FACE('',(#2619),#1589,.T.);
#22359=ADVANCED_FACE('',(#2620),#1590,.F.);
#22360=ADVANCED_FACE('',(#2621),#1591,.F.);
#22361=ADVANCED_FACE('',(#2622),#1592,.F.);
#22362=ADVANCED_FACE('',(#2623),#1593,.T.);
#22363=ADVANCED_FACE('',(#2624),#1594,.F.);
#22364=ADVANCED_FACE('',(#2625),#1595,.F.);
#22365=ADVANCED_FACE('',(#2626),#1596,.F.);
#22366=ADVANCED_FACE('',(#2627),#1597,.T.);
#22367=ADVANCED_FACE('',(#2628),#1598,.F.);
#22368=ADVANCED_FACE('',(#2629),#1599,.F.);
#22369=ADVANCED_FACE('',(#2630),#1600,.F.);
#22370=ADVANCED_FACE('',(#2631),#1601,.T.);
#22371=ADVANCED_FACE('',(#2632),#1602,.F.);
#22372=ADVANCED_FACE('',(#2633),#1603,.F.);
#22373=ADVANCED_FACE('',(#2634),#1604,.F.);
#22374=ADVANCED_FACE('',(#2635),#1605,.T.);
#22375=ADVANCED_FACE('',(#2636),#1606,.F.);
#22376=ADVANCED_FACE('',(#2637),#1607,.F.);
#22377=ADVANCED_FACE('',(#2638),#1608,.F.);
#22378=ADVANCED_FACE('',(#2639),#1609,.T.);
#22379=ADVANCED_FACE('',(#2640),#1610,.F.);
#22380=ADVANCED_FACE('',(#2641),#1611,.F.);
#22381=ADVANCED_FACE('',(#2642),#1612,.F.);
#22382=ADVANCED_FACE('',(#2643),#1613,.T.);
#22383=ADVANCED_FACE('',(#2644),#1614,.F.);
#22384=ADVANCED_FACE('',(#2645),#1615,.F.);
#22385=ADVANCED_FACE('',(#2646),#1616,.F.);
#22386=ADVANCED_FACE('',(#2647),#1617,.T.);
#22387=ADVANCED_FACE('',(#2648),#1618,.F.);
#22388=ADVANCED_FACE('',(#2649),#1619,.F.);
#22389=ADVANCED_FACE('',(#2650),#1620,.F.);
#22390=ADVANCED_FACE('',(#2651),#1621,.T.);
#22391=ADVANCED_FACE('',(#2652),#1622,.F.);
#22392=ADVANCED_FACE('',(#2653),#1623,.F.);
#22393=ADVANCED_FACE('',(#2654),#1624,.F.);
#22394=ADVANCED_FACE('',(#2655),#1625,.T.);
#22395=ADVANCED_FACE('',(#2656),#1626,.F.);
#22396=ADVANCED_FACE('',(#2657),#1627,.F.);
#22397=ADVANCED_FACE('',(#2658),#1628,.F.);
#22398=ADVANCED_FACE('',(#2659),#1629,.T.);
#22399=ADVANCED_FACE('',(#2660),#1630,.F.);
#22400=ADVANCED_FACE('',(#2661),#1631,.F.);
#22401=ADVANCED_FACE('',(#2662),#1632,.F.);
#22402=ADVANCED_FACE('',(#2663),#1633,.T.);
#22403=ADVANCED_FACE('',(#2664),#1634,.F.);
#22404=ADVANCED_FACE('',(#2665),#1635,.F.);
#22405=ADVANCED_FACE('',(#2666),#1636,.F.);
#22406=ADVANCED_FACE('',(#2667),#1637,.T.);
#22407=ADVANCED_FACE('',(#2668),#1638,.F.);
#22408=ADVANCED_FACE('',(#2669),#1639,.F.);
#22409=ADVANCED_FACE('',(#2670),#1640,.F.);
#22410=ADVANCED_FACE('',(#2671),#1641,.T.);
#22411=ADVANCED_FACE('',(#2672),#1642,.F.);
#22412=ADVANCED_FACE('',(#2673),#1643,.F.);
#22413=ADVANCED_FACE('',(#2674),#1644,.F.);
#22414=ADVANCED_FACE('',(#2675),#1645,.T.);
#22415=ADVANCED_FACE('',(#2676),#1646,.F.);
#22416=ADVANCED_FACE('',(#2677),#1647,.F.);
#22417=ADVANCED_FACE('',(#2678),#1648,.F.);
#22418=ADVANCED_FACE('',(#2679),#1649,.T.);
#22419=ADVANCED_FACE('',(#2680),#1026,.T.);
#22420=ADVANCED_FACE('',(#2681),#21936,.T.);
#22421=ADVANCED_FACE('',(#2682),#1650,.T.);
#22422=ADVANCED_FACE('',(#2683,#1345),#1651,.F.);
#22423=ADVANCED_FACE('',(#2684),#1027,.F.);
#22424=ADVANCED_FACE('',(#2685,#1346,#1347,#1348,#1349,#1350,#1351,#1352,
#1353,#1354,#1355,#1356,#1357,#1358,#1359,#1360,#1361,#1362,#1363,#1364,
#1365,#1366,#1367,#1368),#1028,.T.);
#22425=ADVANCED_FACE('',(#2686,#1369),#1652,.T.);
#22426=ADVANCED_FACE('',(#2687),#1029,.T.);
#22427=ADVANCED_FACE('',(#2688),#21937,.T.);
#22428=ADVANCED_FACE('',(#2689,#1370),#1653,.T.);
#22429=ADVANCED_FACE('',(#2690),#1654,.T.);
#22430=ADVANCED_FACE('',(#2691),#1655,.T.);
#22431=ADVANCED_FACE('',(#2692),#1656,.T.);
#22432=ADVANCED_FACE('',(#2693),#1657,.T.);
#22433=ADVANCED_FACE('',(#2694),#1658,.T.);
#22434=ADVANCED_FACE('',(#2695),#1659,.T.);
#22435=ADVANCED_FACE('',(#2696,#1371),#1660,.T.);
#22436=ADVANCED_FACE('',(#2697,#1372,#1373,#1374,#1375,#1376),#1661,.F.);
#22437=ADVANCED_FACE('',(#2698),#1662,.T.);
#22438=ADVANCED_FACE('',(#2699),#1663,.T.);
#22439=ADVANCED_FACE('',(#2700),#1664,.T.);
#22440=ADVANCED_FACE('',(#2701),#1665,.T.);
#22441=ADVANCED_FACE('',(#2702,#1377,#1378,#1379,#1380,#1381),#1666,.T.);
#22442=ADVANCED_FACE('',(#2703),#1667,.T.);
#22443=ADVANCED_FACE('',(#2704),#21938,.T.);
#22444=ADVANCED_FACE('',(#2705),#1030,.T.);
#23308=CLOSED_SHELL('',(#22294,#22295,#22296,#22297,#22298,#22299,#22300,
#22301,#22302,#22303,#22304,#22305,#22306,#22307,#22308,#22309,#22310,#22311,
#22312,#22313,#22314,#22315,#22316,#22317,#22318,#22319,#22320,#22321,#22322,
#22323,#22324,#22325,#22326,#22327,#22328,#22329,#22330,#22331,#22332,#22333,
#22334,#22335,#22336,#22337,#22338,#22339,#22340,#22341,#22342,#22343,#22344,
#22345,#22346,#22347,#22348,#22349,#22350,#22351,#22352,#22353,#22354,#22355,
#22356,#22357,#22358,#22359,#22360,#22361,#22362,#22363,#22364,#22365,#22366,
#22367,#22368,#22369,#22370,#22371,#22372,#22373,#22374,#22375,#22376,#22377,
#22378,#22379,#22380,#22381,#22382,#22383,#22384,#22385,#22386,#22387,#22388,
#22389,#22390,#22391,#22392,#22393,#22394,#22395,#22396,#22397,#22398,#22399,
#22400,#22401,#22402,#22403,#22404,#22405,#22406,#22407,#22408,#22409,#22410,
#22411,#22412,#22413,#22414,#22415,#22416,#22417,#22418,#22419,#22420,#22421,
#22422,#22423,#22424,#22425,#22426,#22427,#22428,#22429,#22430,#22431,#22432,
#22433,#22434,#22435,#22436,#22437,#22438,#22439,#22440,#22441,#22442,#22443,
#22444));
#24107=AXIS2_PLACEMENT_3D('',#33233,#27280,#27281);
#24108=AXIS2_PLACEMENT_3D('',#33234,#27282,#27283);
#24109=AXIS2_PLACEMENT_3D('',#33266,#27286,#27287);
#24110=AXIS2_PLACEMENT_3D('',#33273,#27288,#27289);
#24111=AXIS2_PLACEMENT_3D('',#33296,#27290,#27291);
#24112=AXIS2_PLACEMENT_3D('',#33344,#27293,#27294);
#24113=AXIS2_PLACEMENT_3D('',#33392,#27296,#27297);
#24114=AXIS2_PLACEMENT_3D('',#33440,#27299,#27300);
#24115=AXIS2_PLACEMENT_3D('',#33488,#27302,#27303);
#24116=AXIS2_PLACEMENT_3D('',#33542,#27305,#27306);
#24117=AXIS2_PLACEMENT_3D('',#33590,#27308,#27309);
#24118=AXIS2_PLACEMENT_3D('',#33638,#27311,#27312);
#24119=AXIS2_PLACEMENT_3D('',#33692,#27314,#27315);
#24120=AXIS2_PLACEMENT_3D('',#33740,#27317,#27318);
#24121=AXIS2_PLACEMENT_3D('',#33751,#27320,#27321);
#24122=AXIS2_PLACEMENT_3D('',#33756,#27322,#27323);
#24123=AXIS2_PLACEMENT_3D('',#33780,#27325,#27326);
#24124=AXIS2_PLACEMENT_3D('',#33805,#27328,#27329);
#24125=AXIS2_PLACEMENT_3D('',#33830,#27331,#27332);
#24126=AXIS2_PLACEMENT_3D('',#33854,#27334,#27335);
#24127=AXIS2_PLACEMENT_3D('',#33879,#27337,#27338);
#24128=AXIS2_PLACEMENT_3D('',#33904,#27340,#27341);
#24129=AXIS2_PLACEMENT_3D('',#33928,#27343,#27344);
#24130=AXIS2_PLACEMENT_3D('',#33954,#27346,#27347);
#24131=AXIS2_PLACEMENT_3D('',#33978,#27349,#27350);
#24132=AXIS2_PLACEMENT_3D('',#34446,#27352,#27353);
#24133=AXIS2_PLACEMENT_3D('',#34509,#27354,#27355);
#24134=AXIS2_PLACEMENT_3D('',#34510,#27356,#27357);
#24135=AXIS2_PLACEMENT_3D('',#34887,#27358,#27359);
#24136=AXIS2_PLACEMENT_3D('',#34889,#27360,#27361);
#24137=AXIS2_PLACEMENT_3D('',#34892,#27363,#27364);
#24138=AXIS2_PLACEMENT_3D('',#34893,#27365,#27366);
#24139=AXIS2_PLACEMENT_3D('',#34895,#27367,#27368);
#24140=AXIS2_PLACEMENT_3D('',#34898,#27370,#27371);
#24141=AXIS2_PLACEMENT_3D('',#34899,#27372,#27373);
#24142=AXIS2_PLACEMENT_3D('',#34901,#27374,#27375);
#24143=AXIS2_PLACEMENT_3D('',#34904,#27377,#27378);
#24144=AXIS2_PLACEMENT_3D('',#34905,#27379,#27380);
#24145=AXIS2_PLACEMENT_3D('',#34907,#27381,#27382);
#24146=AXIS2_PLACEMENT_3D('',#34910,#27384,#27385);
#24147=AXIS2_PLACEMENT_3D('',#34911,#27386,#27387);
#24148=AXIS2_PLACEMENT_3D('',#34920,#27392,#27393);
#24149=AXIS2_PLACEMENT_3D('',#34922,#27394,#27395);
#24150=AXIS2_PLACEMENT_3D('',#34924,#27397,#27398);
#24151=AXIS2_PLACEMENT_3D('',#34928,#27401,#27402);
#24152=AXIS2_PLACEMENT_3D('',#34929,#27403,#27404);
#24153=AXIS2_PLACEMENT_3D('',#34930,#27405,#27406);
#24154=AXIS2_PLACEMENT_3D('',#34939,#27411,#27412);
#24155=AXIS2_PLACEMENT_3D('',#34941,#27413,#27414);
#24156=AXIS2_PLACEMENT_3D('',#34943,#27416,#27417);
#24157=AXIS2_PLACEMENT_3D('',#34947,#27420,#27421);
#24158=AXIS2_PLACEMENT_3D('',#34948,#27422,#27423);
#24159=AXIS2_PLACEMENT_3D('',#34949,#27424,#27425);
#24160=AXIS2_PLACEMENT_3D('',#34958,#27430,#27431);
#24161=AXIS2_PLACEMENT_3D('',#34960,#27432,#27433);
#24162=AXIS2_PLACEMENT_3D('',#34962,#27435,#27436);
#24163=AXIS2_PLACEMENT_3D('',#34966,#27439,#27440);
#24164=AXIS2_PLACEMENT_3D('',#34967,#27441,#27442);
#24165=AXIS2_PLACEMENT_3D('',#34968,#27443,#27444);
#24166=AXIS2_PLACEMENT_3D('',#34977,#27449,#27450);
#24167=AXIS2_PLACEMENT_3D('',#34979,#27451,#27452);
#24168=AXIS2_PLACEMENT_3D('',#34981,#27454,#27455);
#24169=AXIS2_PLACEMENT_3D('',#34985,#27458,#27459);
#24170=AXIS2_PLACEMENT_3D('',#34986,#27460,#27461);
#24171=AXIS2_PLACEMENT_3D('',#34987,#27462,#27463);
#24172=AXIS2_PLACEMENT_3D('',#34996,#27468,#27469);
#24173=AXIS2_PLACEMENT_3D('',#34998,#27470,#27471);
#24174=AXIS2_PLACEMENT_3D('',#35000,#27473,#27474);
#24175=AXIS2_PLACEMENT_3D('',#35004,#27477,#27478);
#24176=AXIS2_PLACEMENT_3D('',#35005,#27479,#27480);
#24177=AXIS2_PLACEMENT_3D('',#35006,#27481,#27482);
#24178=AXIS2_PLACEMENT_3D('',#35015,#27487,#27488);
#24179=AXIS2_PLACEMENT_3D('',#35017,#27489,#27490);
#24180=AXIS2_PLACEMENT_3D('',#35019,#27492,#27493);
#24181=AXIS2_PLACEMENT_3D('',#35023,#27496,#27497);
#24182=AXIS2_PLACEMENT_3D('',#35024,#27498,#27499);
#24183=AXIS2_PLACEMENT_3D('',#35025,#27500,#27501);
#24184=AXIS2_PLACEMENT_3D('',#35034,#27506,#27507);
#24185=AXIS2_PLACEMENT_3D('',#35036,#27508,#27509);
#24186=AXIS2_PLACEMENT_3D('',#35038,#27511,#27512);
#24187=AXIS2_PLACEMENT_3D('',#35042,#27515,#27516);
#24188=AXIS2_PLACEMENT_3D('',#35043,#27517,#27518);
#24189=AXIS2_PLACEMENT_3D('',#35044,#27519,#27520);
#24190=AXIS2_PLACEMENT_3D('',#35053,#27525,#27526);
#24191=AXIS2_PLACEMENT_3D('',#35055,#27527,#27528);
#24192=AXIS2_PLACEMENT_3D('',#35057,#27530,#27531);
#24193=AXIS2_PLACEMENT_3D('',#35061,#27534,#27535);
#24194=AXIS2_PLACEMENT_3D('',#35062,#27536,#27537);
#24195=AXIS2_PLACEMENT_3D('',#35063,#27538,#27539);
#24196=AXIS2_PLACEMENT_3D('',#35072,#27544,#27545);
#24197=AXIS2_PLACEMENT_3D('',#35074,#27546,#27547);
#24198=AXIS2_PLACEMENT_3D('',#35076,#27549,#27550);
#24199=AXIS2_PLACEMENT_3D('',#35080,#27553,#27554);
#24200=AXIS2_PLACEMENT_3D('',#35081,#27555,#27556);
#24201=AXIS2_PLACEMENT_3D('',#35082,#27557,#27558);
#24202=AXIS2_PLACEMENT_3D('',#35091,#27563,#27564);
#24203=AXIS2_PLACEMENT_3D('',#35093,#27565,#27566);
#24204=AXIS2_PLACEMENT_3D('',#35095,#27568,#27569);
#24205=AXIS2_PLACEMENT_3D('',#35099,#27572,#27573);
#24206=AXIS2_PLACEMENT_3D('',#35100,#27574,#27575);
#24207=AXIS2_PLACEMENT_3D('',#35101,#27576,#27577);
#24208=AXIS2_PLACEMENT_3D('',#35110,#27582,#27583);
#24209=AXIS2_PLACEMENT_3D('',#35112,#27584,#27585);
#24210=AXIS2_PLACEMENT_3D('',#35114,#27587,#27588);
#24211=AXIS2_PLACEMENT_3D('',#35118,#27591,#27592);
#24212=AXIS2_PLACEMENT_3D('',#35119,#27593,#27594);
#24213=AXIS2_PLACEMENT_3D('',#35120,#27595,#27596);
#24214=AXIS2_PLACEMENT_3D('',#35129,#27601,#27602);
#24215=AXIS2_PLACEMENT_3D('',#35131,#27603,#27604);
#24216=AXIS2_PLACEMENT_3D('',#35134,#27606,#27607);
#24217=AXIS2_PLACEMENT_3D('',#35135,#27608,#27609);
#24218=AXIS2_PLACEMENT_3D('',#35139,#27612,#27613);
#24219=AXIS2_PLACEMENT_3D('',#35141,#27614,#27615);
#24220=AXIS2_PLACEMENT_3D('',#35142,#27616,#27617);
#24221=AXIS2_PLACEMENT_3D('',#35143,#27618,#27619);
#24222=AXIS2_PLACEMENT_3D('',#35152,#27624,#27625);
#24223=AXIS2_PLACEMENT_3D('',#35154,#27626,#27627);
#24224=AXIS2_PLACEMENT_3D('',#35156,#27629,#27630);
#24225=AXIS2_PLACEMENT_3D('',#35160,#27633,#27634);
#24226=AXIS2_PLACEMENT_3D('',#35161,#27635,#27636);
#24227=AXIS2_PLACEMENT_3D('',#35162,#27637,#27638);
#24228=AXIS2_PLACEMENT_3D('',#35171,#27643,#27644);
#24229=AXIS2_PLACEMENT_3D('',#35173,#27645,#27646);
#24230=AXIS2_PLACEMENT_3D('',#35175,#27648,#27649);
#24231=AXIS2_PLACEMENT_3D('',#35179,#27652,#27653);
#24232=AXIS2_PLACEMENT_3D('',#35180,#27654,#27655);
#24233=AXIS2_PLACEMENT_3D('',#35181,#27656,#27657);
#24234=AXIS2_PLACEMENT_3D('',#35190,#27662,#27663);
#24235=AXIS2_PLACEMENT_3D('',#35192,#27664,#27665);
#24236=AXIS2_PLACEMENT_3D('',#35194,#27667,#27668);
#24237=AXIS2_PLACEMENT_3D('',#35198,#27671,#27672);
#24238=AXIS2_PLACEMENT_3D('',#35199,#27673,#27674);
#24239=AXIS2_PLACEMENT_3D('',#35200,#27675,#27676);
#24240=AXIS2_PLACEMENT_3D('',#35209,#27681,#27682);
#24241=AXIS2_PLACEMENT_3D('',#35211,#27683,#27684);
#24242=AXIS2_PLACEMENT_3D('',#35213,#27686,#27687);
#24243=AXIS2_PLACEMENT_3D('',#35217,#27690,#27691);
#24244=AXIS2_PLACEMENT_3D('',#35218,#27692,#27693);
#24245=AXIS2_PLACEMENT_3D('',#35219,#27694,#27695);
#24246=AXIS2_PLACEMENT_3D('',#35228,#27700,#27701);
#24247=AXIS2_PLACEMENT_3D('',#35230,#27702,#27703);
#24248=AXIS2_PLACEMENT_3D('',#35232,#27705,#27706);
#24249=AXIS2_PLACEMENT_3D('',#35236,#27709,#27710);
#24250=AXIS2_PLACEMENT_3D('',#35237,#27711,#27712);
#24251=AXIS2_PLACEMENT_3D('',#35238,#27713,#27714);
#24252=AXIS2_PLACEMENT_3D('',#35247,#27719,#27720);
#24253=AXIS2_PLACEMENT_3D('',#35249,#27721,#27722);
#24254=AXIS2_PLACEMENT_3D('',#35251,#27724,#27725);
#24255=AXIS2_PLACEMENT_3D('',#35255,#27728,#27729);
#24256=AXIS2_PLACEMENT_3D('',#35256,#27730,#27731);
#24257=AXIS2_PLACEMENT_3D('',#35257,#27732,#27733);
#24258=AXIS2_PLACEMENT_3D('',#35266,#27738,#27739);
#24259=AXIS2_PLACEMENT_3D('',#35268,#27740,#27741);
#24260=AXIS2_PLACEMENT_3D('',#35270,#27743,#27744);
#24261=AXIS2_PLACEMENT_3D('',#35274,#27747,#27748);
#24262=AXIS2_PLACEMENT_3D('',#35275,#27749,#27750);
#24263=AXIS2_PLACEMENT_3D('',#35276,#27751,#27752);
#24264=AXIS2_PLACEMENT_3D('',#35285,#27757,#27758);
#24265=AXIS2_PLACEMENT_3D('',#35287,#27759,#27760);
#24266=AXIS2_PLACEMENT_3D('',#35289,#27762,#27763);
#24267=AXIS2_PLACEMENT_3D('',#35293,#27766,#27767);
#24268=AXIS2_PLACEMENT_3D('',#35294,#27768,#27769);
#24269=AXIS2_PLACEMENT_3D('',#35295,#27770,#27771);
#24270=AXIS2_PLACEMENT_3D('',#35304,#27776,#27777);
#24271=AXIS2_PLACEMENT_3D('',#35306,#27778,#27779);
#24272=AXIS2_PLACEMENT_3D('',#35308,#27781,#27782);
#24273=AXIS2_PLACEMENT_3D('',#35312,#27785,#27786);
#24274=AXIS2_PLACEMENT_3D('',#35313,#27787,#27788);
#24275=AXIS2_PLACEMENT_3D('',#35314,#27789,#27790);
#24276=AXIS2_PLACEMENT_3D('',#35323,#27795,#27796);
#24277=AXIS2_PLACEMENT_3D('',#35325,#27797,#27798);
#24278=AXIS2_PLACEMENT_3D('',#35327,#27800,#27801);
#24279=AXIS2_PLACEMENT_3D('',#35331,#27804,#27805);
#24280=AXIS2_PLACEMENT_3D('',#35332,#27806,#27807);
#24281=AXIS2_PLACEMENT_3D('',#35333,#27808,#27809);
#24282=AXIS2_PLACEMENT_3D('',#35342,#27814,#27815);
#24283=AXIS2_PLACEMENT_3D('',#35344,#27816,#27817);
#24284=AXIS2_PLACEMENT_3D('',#35346,#27819,#27820);
#24285=AXIS2_PLACEMENT_3D('',#35350,#27823,#27824);
#24286=AXIS2_PLACEMENT_3D('',#35351,#27825,#27826);
#24287=AXIS2_PLACEMENT_3D('',#35352,#27827,#27828);
#24288=AXIS2_PLACEMENT_3D('',#35361,#27833,#27834);
#24289=AXIS2_PLACEMENT_3D('',#35363,#27835,#27836);
#24290=AXIS2_PLACEMENT_3D('',#35365,#27838,#27839);
#24291=AXIS2_PLACEMENT_3D('',#35369,#27842,#27843);
#24292=AXIS2_PLACEMENT_3D('',#35370,#27844,#27845);
#24293=AXIS2_PLACEMENT_3D('',#35371,#27846,#27847);
#24294=AXIS2_PLACEMENT_3D('',#35373,#27848,#27849);
#24295=AXIS2_PLACEMENT_3D('',#35376,#27851,#27852);
#24296=AXIS2_PLACEMENT_3D('',#35377,#27853,#27854);
#24297=AXIS2_PLACEMENT_3D('',#35379,#27855,#27856);
#24298=AXIS2_PLACEMENT_3D('',#35381,#27858,#27859);
#24299=AXIS2_PLACEMENT_3D('',#35382,#27860,#27861);
#24300=AXIS2_PLACEMENT_3D('',#35384,#27862,#27863);
#24301=AXIS2_PLACEMENT_3D('',#35385,#27864,#27865);
#24302=AXIS2_PLACEMENT_3D('',#35388,#27867,#27868);
#24303=AXIS2_PLACEMENT_3D('',#35389,#27869,#27870);
#24304=AXIS2_PLACEMENT_3D('',#35391,#27871,#27872);
#24305=AXIS2_PLACEMENT_3D('',#35395,#27875,#27876);
#24306=AXIS2_PLACEMENT_3D('',#35396,#27877,#27878);
#24307=AXIS2_PLACEMENT_3D('',#35398,#27879,#27880);
#24308=AXIS2_PLACEMENT_3D('',#35399,#27881,#27882);
#24309=AXIS2_PLACEMENT_3D('',#35401,#27883,#27884);
#24310=AXIS2_PLACEMENT_3D('',#35403,#27886,#27887);
#24311=AXIS2_PLACEMENT_3D('',#35405,#27888,#27889);
#24312=AXIS2_PLACEMENT_3D('',#35407,#27891,#27892);
#24313=AXIS2_PLACEMENT_3D('',#35408,#27893,#27894);
#24314=AXIS2_PLACEMENT_3D('',#35417,#27899,#27900);
#24315=AXIS2_PLACEMENT_3D('',#35423,#27904,#27905);
#24316=AXIS2_PLACEMENT_3D('',#35429,#27909,#27910);
#24317=AXIS2_PLACEMENT_3D('',#35435,#27914,#27915);
#24318=AXIS2_PLACEMENT_3D('',#35441,#27919,#27920);
#24319=AXIS2_PLACEMENT_3D('',#35444,#27923,#27924);
#24320=AXIS2_PLACEMENT_3D('',#35445,#27925,#27926);
#24321=AXIS2_PLACEMENT_3D('',#35454,#27931,#27932);
#24322=AXIS2_PLACEMENT_3D('',#35455,#27933,#27934);
#24323=AXIS2_PLACEMENT_3D('',#35461,#27938,#27939);
#24324=AXIS2_PLACEMENT_3D('',#35465,#27942,#27943);
#24325=AXIS2_PLACEMENT_3D('',#35469,#27946,#27947);
#24326=AXIS2_PLACEMENT_3D('',#35471,#27949,#27950);
#24327=AXIS2_PLACEMENT_3D('',#35472,#27951,#27952);
#24328=AXIS2_PLACEMENT_3D('',#35474,#27953,#27954);
#24329=AXIS2_PLACEMENT_3D('',#35475,#27955,#27956);
#24330=AXIS2_PLACEMENT_3D('',#35477,#27958,#27959);
#27280=DIRECTION('axis',(0.,0.,1.));
#27281=DIRECTION('refdir',(1.,0.,0.));
#27282=DIRECTION('center_axis',(0.,0.,1.));
#27283=DIRECTION('ref_axis',(1.,0.,0.));
#27284=DIRECTION('',(0.,0.,-1.));
#27285=DIRECTION('',(0.,0.,-1.));
#27286=DIRECTION('center_axis',(0.,0.,1.));
#27287=DIRECTION('ref_axis',(1.,0.,0.));
#27288=DIRECTION('center_axis',(0.,0.,-1.));
#27289=DIRECTION('ref_axis',(1.,0.,0.));
#27290=DIRECTION('center_axis',(0.,0.,1.));
#27291=DIRECTION('ref_axis',(1.,0.,0.));
#27292=DIRECTION('',(0.,0.,-1.));
#27293=DIRECTION('center_axis',(0.,0.,1.));
#27294=DIRECTION('ref_axis',(1.,0.,0.));
#27295=DIRECTION('',(0.,0.,-1.));
#27296=DIRECTION('center_axis',(0.,0.,1.));
#27297=DIRECTION('ref_axis',(1.,0.,0.));
#27298=DIRECTION('',(0.,0.,-1.));
#27299=DIRECTION('center_axis',(0.,0.,1.));
#27300=DIRECTION('ref_axis',(1.,0.,0.));
#27301=DIRECTION('',(0.,0.,-1.));
#27302=DIRECTION('center_axis',(0.,0.,1.));
#27303=DIRECTION('ref_axis',(1.,0.,0.));
#27304=DIRECTION('',(0.,0.,-1.));
#27305=DIRECTION('center_axis',(0.,0.,1.));
#27306=DIRECTION('ref_axis',(1.,0.,0.));
#27307=DIRECTION('',(0.,0.,-1.));
#27308=DIRECTION('center_axis',(0.,0.,1.));
#27309=DIRECTION('ref_axis',(1.,0.,0.));
#27310=DIRECTION('',(0.,0.,-1.));
#27311=DIRECTION('center_axis',(0.,0.,1.));
#27312=DIRECTION('ref_axis',(1.,0.,0.));
#27313=DIRECTION('',(0.,0.,-1.));
#27314=DIRECTION('center_axis',(0.,0.,1.));
#27315=DIRECTION('ref_axis',(1.,0.,0.));
#27316=DIRECTION('',(0.,0.,-1.));
#27317=DIRECTION('center_axis',(0.,0.,1.));
#27318=DIRECTION('ref_axis',(1.,5.20993371284765E-14,0.));
#27319=DIRECTION('',(0.,0.,1.));
#27320=DIRECTION('center_axis',(0.,0.,1.));
#27321=DIRECTION('ref_axis',(1.,5.20993371284765E-14,0.));
#27322=DIRECTION('center_axis',(0.,0.,1.));
#27323=DIRECTION('ref_axis',(1.,5.20993371284765E-14,0.));
#27324=DIRECTION('',(0.,0.,1.));
#27325=DIRECTION('center_axis',(0.,0.,1.));
#27326=DIRECTION('ref_axis',(1.,5.20993371284765E-14,0.));
#27327=DIRECTION('',(0.,0.,1.));
#27328=DIRECTION('center_axis',(0.,0.,1.));
#27329=DIRECTION('ref_axis',(1.,5.20993371284765E-14,0.));
#27330=DIRECTION('',(0.,0.,1.));
#27331=DIRECTION('center_axis',(0.,0.,1.));
#27332=DIRECTION('ref_axis',(1.,5.20993371284765E-14,0.));
#27333=DIRECTION('',(0.,0.,1.));
#27334=DIRECTION('center_axis',(0.,0.,1.));
#27335=DIRECTION('ref_axis',(1.,5.20993371284765E-14,0.));
#27336=DIRECTION('',(0.,0.,1.));
#27337=DIRECTION('center_axis',(0.,0.,1.));
#27338=DIRECTION('ref_axis',(1.,5.20993371284765E-14,0.));
#27339=DIRECTION('',(0.,0.,1.));
#27340=DIRECTION('center_axis',(0.,0.,1.));
#27341=DIRECTION('ref_axis',(1.,5.20993371284765E-14,0.));
#27342=DIRECTION('',(0.,0.,1.));
#27343=DIRECTION('center_axis',(0.,0.,1.));
#27344=DIRECTION('ref_axis',(1.,5.20993371284765E-14,0.));
#27345=DIRECTION('',(0.,0.,1.));
#27346=DIRECTION('center_axis',(0.,0.,1.));
#27347=DIRECTION('ref_axis',(1.,5.20993371284765E-14,0.));
#27348=DIRECTION('',(0.,0.,1.));
#27349=DIRECTION('center_axis',(0.,0.,1.));
#27350=DIRECTION('ref_axis',(1.,5.20993371284765E-14,0.));
#27351=DIRECTION('',(0.,0.,1.));
#27352=DIRECTION('center_axis',(0.,0.,1.));
#27353=DIRECTION('ref_axis',(1.,0.,0.));
#27354=DIRECTION('center_axis',(0.,0.,-1.));
#27355=DIRECTION('ref_axis',(1.,5.20993371284765E-14,0.));
#27356=DIRECTION('center_axis',(0.,0.,1.));
#27357=DIRECTION('ref_axis',(0.464898683733536,0.885363887823998,0.));
#27358=DIRECTION('center_axis',(0.,0.,1.));
#27359=DIRECTION('ref_axis',(1.,0.,0.));
#27360=DIRECTION('center_axis',(0.,0.,1.));
#27361=DIRECTION('ref_axis',(1.,0.,0.));
#27362=DIRECTION('',(0.,0.,1.));
#27363=DIRECTION('center_axis',(0.,0.,-1.));
#27364=DIRECTION('ref_axis',(1.,0.,0.));
#27365=DIRECTION('center_axis',(0.,0.,1.));
#27366=DIRECTION('ref_axis',(1.,0.,0.));
#27367=DIRECTION('center_axis',(0.,0.,1.));
#27368=DIRECTION('ref_axis',(1.,0.,0.));
#27369=DIRECTION('',(0.,0.,1.));
#27370=DIRECTION('center_axis',(0.,0.,-1.));
#27371=DIRECTION('ref_axis',(1.,0.,0.));
#27372=DIRECTION('center_axis',(0.,0.,1.));
#27373=DIRECTION('ref_axis',(1.,0.,0.));
#27374=DIRECTION('center_axis',(0.,0.,1.));
#27375=DIRECTION('ref_axis',(1.,0.,0.));
#27376=DIRECTION('',(0.,0.,1.));
#27377=DIRECTION('center_axis',(0.,0.,-1.));
#27378=DIRECTION('ref_axis',(1.,0.,0.));
#27379=DIRECTION('center_axis',(0.,0.,1.));
#27380=DIRECTION('ref_axis',(1.,0.,0.));
#27381=DIRECTION('center_axis',(0.,0.,1.));
#27382=DIRECTION('ref_axis',(1.,0.,0.));
#27383=DIRECTION('',(0.,0.,1.));
#27384=DIRECTION('center_axis',(0.,0.,-1.));
#27385=DIRECTION('ref_axis',(1.,0.,0.));
#27386=DIRECTION('center_axis',(-0.718878223686824,-0.695136029499893,0.));
#27387=DIRECTION('ref_axis',(0.695136029499893,-0.718878223686824,0.));
#27388=DIRECTION('',(0.,0.,1.));
#27389=DIRECTION('',(0.695136029499893,-0.718878223686824,0.));
#27390=DIRECTION('',(0.,0.,1.));
#27391=DIRECTION('',(0.695136029499893,-0.718878223686824,0.));
#27392=DIRECTION('center_axis',(0.,0.,1.));
#27393=DIRECTION('ref_axis',(0.965925826289068,-0.258819045102522,0.));
#27394=DIRECTION('center_axis',(0.,0.,1.));
#27395=DIRECTION('ref_axis',(1.,0.,0.));
#27396=DIRECTION('',(-0.961444572476169,-0.274998789190274,0.));
#27397=DIRECTION('center_axis',(-0.274998789190274,0.961444572476169,0.));
#27398=DIRECTION('ref_axis',(-0.961444572476169,-0.274998789190274,0.));
#27399=DIRECTION('',(0.,0.,-1.));
#27400=DIRECTION('',(-0.961444572476169,-0.274998789190274,0.));
#27401=DIRECTION('center_axis',(0.,0.,1.));
#27402=DIRECTION('ref_axis',(0.965925826289068,-0.258819045102522,0.));
#27403=DIRECTION('center_axis',(0.,0.,-1.));
#27404=DIRECTION('ref_axis',(1.,0.,0.));
#27405=DIRECTION('center_axis',(-0.874297485587433,-0.485390468278367,0.));
#27406=DIRECTION('ref_axis',(0.485390468278367,-0.874297485587433,0.));
#27407=DIRECTION('',(0.,0.,1.));
#27408=DIRECTION('',(0.485390468278367,-0.874297485587433,0.));
#27409=DIRECTION('',(0.,0.,1.));
#27410=DIRECTION('',(0.485390468278367,-0.874297485587433,0.));
#27411=DIRECTION('center_axis',(0.,0.,1.));
#27412=DIRECTION('ref_axis',(0.866025403784438,-0.500000000000001,0.));
#27413=DIRECTION('center_axis',(0.,0.,1.));
#27414=DIRECTION('ref_axis',(1.,0.,0.));
#27415=DIRECTION('',(-0.99985906712276,-0.0167882665098254,0.));
#27416=DIRECTION('center_axis',(-0.0167882665098254,0.99985906712276,0.));
#27417=DIRECTION('ref_axis',(-0.99985906712276,-0.0167882665098254,0.));
#27418=DIRECTION('',(0.,0.,-1.));
#27419=DIRECTION('',(-0.99985906712276,-0.0167882665098254,0.));
#27420=DIRECTION('center_axis',(0.,0.,1.));
#27421=DIRECTION('ref_axis',(0.866025403784438,-0.500000000000001,0.));
#27422=DIRECTION('center_axis',(0.,0.,-1.));
#27423=DIRECTION('ref_axis',(1.,0.,0.));
#27424=DIRECTION('center_axis',(-0.970134818690168,-0.242566348789345,0.));
#27425=DIRECTION('ref_axis',(0.242566348789345,-0.970134818690168,0.));
#27426=DIRECTION('',(0.,0.,1.));
#27427=DIRECTION('',(0.242566348789345,-0.970134818690168,0.));
#27428=DIRECTION('',(0.,0.,1.));
#27429=DIRECTION('',(0.242566348789345,-0.970134818690168,0.));
#27430=DIRECTION('center_axis',(0.,0.,1.));
#27431=DIRECTION('ref_axis',(0.707106781186547,-0.707106781186548,0.));
#27432=DIRECTION('center_axis',(0.,0.,1.));
#27433=DIRECTION('ref_axis',(1.,0.,0.));
#27434=DIRECTION('',(-0.970134818690168,0.242566348789345,0.));
#27435=DIRECTION('center_axis',(0.242566348789345,0.970134818690168,0.));
#27436=DIRECTION('ref_axis',(-0.970134818690168,0.242566348789345,0.));
#27437=DIRECTION('',(0.,0.,-1.));
#27438=DIRECTION('',(-0.970134818690168,0.242566348789345,0.));
#27439=DIRECTION('center_axis',(0.,0.,1.));
#27440=DIRECTION('ref_axis',(0.707106781186547,-0.707106781186548,0.));
#27441=DIRECTION('center_axis',(0.,0.,-1.));
#27442=DIRECTION('ref_axis',(1.,0.,0.));
#27443=DIRECTION('center_axis',(-0.99985906712276,0.0167882665098268,0.));
#27444=DIRECTION('ref_axis',(-0.0167882665098268,-0.99985906712276,0.));
#27445=DIRECTION('',(0.,0.,1.));
#27446=DIRECTION('',(-0.0167882665098268,-0.99985906712276,0.));
#27447=DIRECTION('',(0.,0.,1.));
#27448=DIRECTION('',(-0.0167882665098268,-0.99985906712276,0.));
#27449=DIRECTION('center_axis',(0.,0.,1.));
#27450=DIRECTION('ref_axis',(0.499999999999999,-0.866025403784439,0.));
#27451=DIRECTION('center_axis',(0.,0.,1.));
#27452=DIRECTION('ref_axis',(1.,0.,0.));
#27453=DIRECTION('',(-0.874297485587433,0.485390468278368,0.));
#27454=DIRECTION('center_axis',(0.485390468278368,0.874297485587433,0.));
#27455=DIRECTION('ref_axis',(-0.874297485587433,0.485390468278368,0.));
#27456=DIRECTION('',(0.,0.,-1.));
#27457=DIRECTION('',(-0.874297485587433,0.485390468278368,0.));
#27458=DIRECTION('center_axis',(0.,0.,1.));
#27459=DIRECTION('ref_axis',(0.499999999999999,-0.866025403784439,0.));
#27460=DIRECTION('center_axis',(0.,0.,-1.));
#27461=DIRECTION('ref_axis',(1.,0.,0.));
#27462=DIRECTION('center_axis',(-0.961444572476169,0.274998789190275,0.));
#27463=DIRECTION('ref_axis',(-0.274998789190275,-0.961444572476169,0.));
#27464=DIRECTION('',(0.,0.,1.));
#27465=DIRECTION('',(-0.274998789190275,-0.961444572476169,0.));
#27466=DIRECTION('',(0.,0.,1.));
#27467=DIRECTION('',(-0.274998789190275,-0.961444572476169,0.));
#27468=DIRECTION('center_axis',(0.,0.,1.));
#27469=DIRECTION('ref_axis',(0.25881904510252,-0.965925826289068,0.));
#27470=DIRECTION('center_axis',(0.,0.,1.));
#27471=DIRECTION('ref_axis',(1.,0.,0.));
#27472=DIRECTION('',(-0.718878223686823,0.695136029499894,0.));
#27473=DIRECTION('center_axis',(0.695136029499894,0.718878223686823,0.));
#27474=DIRECTION('ref_axis',(-0.718878223686823,0.695136029499894,0.));
#27475=DIRECTION('',(0.,0.,-1.));
#27476=DIRECTION('',(-0.718878223686823,0.695136029499894,0.));
#27477=DIRECTION('center_axis',(0.,0.,1.));
#27478=DIRECTION('ref_axis',(0.25881904510252,-0.965925826289068,0.));
#27479=DIRECTION('center_axis',(0.,0.,-1.));
#27480=DIRECTION('ref_axis',(1.,0.,0.));
#27481=DIRECTION('center_axis',(-0.857509219077607,0.514468598844393,0.));
#27482=DIRECTION('ref_axis',(-0.514468598844393,-0.857509219077607,0.));
#27483=DIRECTION('',(0.,0.,1.));
#27484=DIRECTION('',(-0.514468598844393,-0.857509219077607,0.));
#27485=DIRECTION('',(0.,0.,1.));
#27486=DIRECTION('',(-0.514468598844393,-0.857509219077607,0.));
#27487=DIRECTION('center_axis',(0.,0.,1.));
#27488=DIRECTION('ref_axis',(-1.94289029309402E-16,-1.,0.));
#27489=DIRECTION('center_axis',(0.,0.,1.));
#27490=DIRECTION('ref_axis',(1.,0.,0.));
#27491=DIRECTION('',(-0.514468598844392,0.857509219077607,0.));
#27492=DIRECTION('center_axis',(0.857509219077607,0.514468598844392,0.));
#27493=DIRECTION('ref_axis',(-0.514468598844392,0.857509219077607,0.));
#27494=DIRECTION('',(0.,0.,-1.));
#27495=DIRECTION('',(-0.514468598844392,0.857509219077607,0.));
#27496=DIRECTION('center_axis',(0.,0.,1.));
#27497=DIRECTION('ref_axis',(-1.94289029309402E-16,-1.,0.));
#27498=DIRECTION('center_axis',(0.,0.,-1.));
#27499=DIRECTION('ref_axis',(1.,0.,0.));
#27500=DIRECTION('center_axis',(-0.695136029499893,0.718878223686824,0.));
#27501=DIRECTION('ref_axis',(-0.718878223686824,-0.695136029499893,0.));
#27502=DIRECTION('',(0.,0.,1.));
#27503=DIRECTION('',(-0.718878223686824,-0.695136029499893,0.));
#27504=DIRECTION('',(0.,0.,1.));
#27505=DIRECTION('',(-0.718878223686824,-0.695136029499893,0.));
#27506=DIRECTION('center_axis',(0.,0.,1.));
#27507=DIRECTION('ref_axis',(-0.258819045102522,-0.965925826289068,0.));
#27508=DIRECTION('center_axis',(0.,0.,1.));
#27509=DIRECTION('ref_axis',(1.,0.,0.));
#27510=DIRECTION('',(-0.274998789190274,0.961444572476169,0.));
#27511=DIRECTION('center_axis',(0.961444572476169,0.274998789190274,0.));
#27512=DIRECTION('ref_axis',(-0.274998789190274,0.961444572476169,0.));
#27513=DIRECTION('',(0.,0.,-1.));
#27514=DIRECTION('',(-0.274998789190274,0.961444572476169,0.));
#27515=DIRECTION('center_axis',(0.,0.,1.));
#27516=DIRECTION('ref_axis',(-0.258819045102522,-0.965925826289068,0.));
#27517=DIRECTION('center_axis',(0.,0.,-1.));
#27518=DIRECTION('ref_axis',(1.,0.,0.));
#27519=DIRECTION('center_axis',(-0.485390468278367,0.874297485587433,0.));
#27520=DIRECTION('ref_axis',(-0.874297485587433,-0.485390468278367,0.));
#27521=DIRECTION('',(0.,0.,1.));
#27522=DIRECTION('',(-0.874297485587433,-0.485390468278367,0.));
#27523=DIRECTION('',(0.,0.,1.));
#27524=DIRECTION('',(-0.874297485587433,-0.485390468278367,0.));
#27525=DIRECTION('center_axis',(0.,0.,1.));
#27526=DIRECTION('ref_axis',(-0.500000000000001,-0.866025403784438,0.));
#27527=DIRECTION('center_axis',(0.,0.,1.));
#27528=DIRECTION('ref_axis',(1.,0.,0.));
#27529=DIRECTION('',(-0.0167882665098254,0.99985906712276,0.));
#27530=DIRECTION('center_axis',(0.99985906712276,0.0167882665098254,0.));
#27531=DIRECTION('ref_axis',(-0.0167882665098254,0.99985906712276,0.));
#27532=DIRECTION('',(0.,0.,-1.));
#27533=DIRECTION('',(-0.0167882665098254,0.99985906712276,0.));
#27534=DIRECTION('center_axis',(0.,0.,1.));
#27535=DIRECTION('ref_axis',(-0.500000000000001,-0.866025403784438,0.));
#27536=DIRECTION('center_axis',(0.,0.,-1.));
#27537=DIRECTION('ref_axis',(1.,0.,0.));
#27538=DIRECTION('center_axis',(-0.242566348789345,0.970134818690168,0.));
#27539=DIRECTION('ref_axis',(-0.970134818690168,-0.242566348789345,0.));
#27540=DIRECTION('',(0.,0.,1.));
#27541=DIRECTION('',(-0.970134818690168,-0.242566348789345,0.));
#27542=DIRECTION('',(0.,0.,1.));
#27543=DIRECTION('',(-0.970134818690168,-0.242566348789345,0.));
#27544=DIRECTION('center_axis',(0.,0.,1.));
#27545=DIRECTION('ref_axis',(-0.707106781186548,-0.707106781186547,0.));
#27546=DIRECTION('center_axis',(0.,0.,1.));
#27547=DIRECTION('ref_axis',(1.,0.,0.));
#27548=DIRECTION('',(0.242566348789346,0.970134818690168,0.));
#27549=DIRECTION('center_axis',(0.970134818690168,-0.242566348789346,0.));
#27550=DIRECTION('ref_axis',(0.242566348789346,0.970134818690168,0.));
#27551=DIRECTION('',(0.,0.,-1.));
#27552=DIRECTION('',(0.242566348789346,0.970134818690168,0.));
#27553=DIRECTION('center_axis',(0.,0.,1.));
#27554=DIRECTION('ref_axis',(-0.707106781186548,-0.707106781186547,0.));
#27555=DIRECTION('center_axis',(0.,0.,-1.));
#27556=DIRECTION('ref_axis',(1.,0.,0.));
#27557=DIRECTION('center_axis',(0.0167882665098262,0.99985906712276,0.));
#27558=DIRECTION('ref_axis',(-0.99985906712276,0.0167882665098262,0.));
#27559=DIRECTION('',(0.,0.,1.));
#27560=DIRECTION('',(-0.99985906712276,0.0167882665098262,0.));
#27561=DIRECTION('',(0.,0.,1.));
#27562=DIRECTION('',(-0.99985906712276,0.0167882665098262,0.));
#27563=DIRECTION('center_axis',(0.,0.,1.));
#27564=DIRECTION('ref_axis',(-0.866025403784439,-0.5,0.));
#27565=DIRECTION('center_axis',(0.,0.,1.));
#27566=DIRECTION('ref_axis',(1.,0.,0.));
#27567=DIRECTION('',(0.485390468278367,0.874297485587433,0.));
#27568=DIRECTION('center_axis',(0.874297485587433,-0.485390468278367,0.));
#27569=DIRECTION('ref_axis',(0.485390468278367,0.874297485587433,0.));
#27570=DIRECTION('',(0.,0.,-1.));
#27571=DIRECTION('',(0.485390468278367,0.874297485587433,0.));
#27572=DIRECTION('center_axis',(0.,0.,1.));
#27573=DIRECTION('ref_axis',(-0.866025403784439,-0.5,0.));
#27574=DIRECTION('center_axis',(0.,0.,-1.));
#27575=DIRECTION('ref_axis',(1.,0.,0.));
#27576=DIRECTION('center_axis',(0.274998789190275,0.961444572476169,0.));
#27577=DIRECTION('ref_axis',(-0.961444572476169,0.274998789190275,0.));
#27578=DIRECTION('',(0.,0.,1.));
#27579=DIRECTION('',(-0.961444572476169,0.274998789190275,0.));
#27580=DIRECTION('',(0.,0.,1.));
#27581=DIRECTION('',(-0.961444572476169,0.274998789190275,0.));
#27582=DIRECTION('center_axis',(0.,0.,1.));
#27583=DIRECTION('ref_axis',(-0.965925826289068,-0.25881904510252,0.));
#27584=DIRECTION('center_axis',(0.,0.,1.));
#27585=DIRECTION('ref_axis',(1.,0.,0.));
#27586=DIRECTION('',(0.695136029499894,0.718878223686823,0.));
#27587=DIRECTION('center_axis',(0.718878223686823,-0.695136029499894,0.));
#27588=DIRECTION('ref_axis',(0.695136029499894,0.718878223686823,0.));
#27589=DIRECTION('',(0.,0.,-1.));
#27590=DIRECTION('',(0.695136029499894,0.718878223686823,0.));
#27591=DIRECTION('center_axis',(0.,0.,1.));
#27592=DIRECTION('ref_axis',(-0.965925826289068,-0.25881904510252,0.));
#27593=DIRECTION('center_axis',(0.,0.,-1.));
#27594=DIRECTION('ref_axis',(1.,0.,0.));
#27595=DIRECTION('center_axis',(0.514468598844393,0.857509219077607,0.));
#27596=DIRECTION('ref_axis',(-0.857509219077607,0.514468598844393,0.));
#27597=DIRECTION('',(0.,0.,1.));
#27598=DIRECTION('',(-0.857509219077607,0.514468598844393,0.));
#27599=DIRECTION('',(0.,0.,1.));
#27600=DIRECTION('',(-0.857509219077607,0.514468598844393,0.));
#27601=DIRECTION('center_axis',(0.,0.,1.));
#27602=DIRECTION('ref_axis',(-1.,1.38777878078145E-16,0.));
#27603=DIRECTION('center_axis',(0.,0.,1.));
#27604=DIRECTION('ref_axis',(1.,0.,0.));
#27605=DIRECTION('',(0.857509219077607,0.514468598844393,0.));
#27606=DIRECTION('center_axis',(0.,0.,1.));
#27607=DIRECTION('ref_axis',(1.,0.,0.));
#27608=DIRECTION('center_axis',(0.514468598844393,-0.857509219077607,0.));
#27609=DIRECTION('ref_axis',(0.857509219077607,0.514468598844393,0.));
#27610=DIRECTION('',(0.,0.,-1.));
#27611=DIRECTION('',(0.857509219077607,0.514468598844393,0.));
#27612=DIRECTION('center_axis',(0.,0.,1.));
#27613=DIRECTION('ref_axis',(-1.,1.38777878078145E-16,0.));
#27614=DIRECTION('center_axis',(0.,0.,-1.));
#27615=DIRECTION('ref_axis',(1.,0.,0.));
#27616=DIRECTION('center_axis',(0.,0.,-1.));
#27617=DIRECTION('ref_axis',(1.,0.,0.));
#27618=DIRECTION('center_axis',(0.718878223686824,0.695136029499894,0.));
#27619=DIRECTION('ref_axis',(-0.695136029499894,0.718878223686824,0.));
#27620=DIRECTION('',(0.,0.,1.));
#27621=DIRECTION('',(-0.695136029499894,0.718878223686824,0.));
#27622=DIRECTION('',(0.,0.,1.));
#27623=DIRECTION('',(-0.695136029499894,0.718878223686824,0.));
#27624=DIRECTION('center_axis',(0.,0.,1.));
#27625=DIRECTION('ref_axis',(-0.965925826289068,0.258819045102521,0.));
#27626=DIRECTION('center_axis',(0.,0.,1.));
#27627=DIRECTION('ref_axis',(1.,0.,0.));
#27628=DIRECTION('',(0.961444572476169,0.274998789190274,0.));
#27629=DIRECTION('center_axis',(0.274998789190274,-0.961444572476169,0.));
#27630=DIRECTION('ref_axis',(0.961444572476169,0.274998789190274,0.));
#27631=DIRECTION('',(0.,0.,-1.));
#27632=DIRECTION('',(0.961444572476169,0.274998789190274,0.));
#27633=DIRECTION('center_axis',(0.,0.,1.));
#27634=DIRECTION('ref_axis',(-0.965925826289068,0.258819045102521,0.));
#27635=DIRECTION('center_axis',(0.,0.,-1.));
#27636=DIRECTION('ref_axis',(1.,0.,0.));
#27637=DIRECTION('center_axis',(0.874297485587433,0.485390468278367,0.));
#27638=DIRECTION('ref_axis',(-0.485390468278367,0.874297485587433,0.));
#27639=DIRECTION('',(0.,0.,1.));
#27640=DIRECTION('',(-0.485390468278367,0.874297485587433,0.));
#27641=DIRECTION('',(0.,0.,1.));
#27642=DIRECTION('',(-0.485390468278367,0.874297485587433,0.));
#27643=DIRECTION('center_axis',(0.,0.,1.));
#27644=DIRECTION('ref_axis',(-0.866025403784438,0.5,0.));
#27645=DIRECTION('center_axis',(0.,0.,1.));
#27646=DIRECTION('ref_axis',(1.,0.,0.));
#27647=DIRECTION('',(0.99985906712276,0.0167882665098256,0.));
#27648=DIRECTION('center_axis',(0.0167882665098256,-0.99985906712276,0.));
#27649=DIRECTION('ref_axis',(0.99985906712276,0.0167882665098256,0.));
#27650=DIRECTION('',(0.,0.,-1.));
#27651=DIRECTION('',(0.99985906712276,0.0167882665098256,0.));
#27652=DIRECTION('center_axis',(0.,0.,1.));
#27653=DIRECTION('ref_axis',(-0.866025403784438,0.5,0.));
#27654=DIRECTION('center_axis',(0.,0.,-1.));
#27655=DIRECTION('ref_axis',(1.,0.,0.));
#27656=DIRECTION('center_axis',(0.970134818690168,0.242566348789345,0.));
#27657=DIRECTION('ref_axis',(-0.242566348789345,0.970134818690168,0.));
#27658=DIRECTION('',(0.,0.,1.));
#27659=DIRECTION('',(-0.242566348789345,0.970134818690168,0.));
#27660=DIRECTION('',(0.,0.,1.));
#27661=DIRECTION('',(-0.242566348789345,0.970134818690168,0.));
#27662=DIRECTION('center_axis',(0.,0.,1.));
#27663=DIRECTION('ref_axis',(-0.707106781186548,0.707106781186548,0.));
#27664=DIRECTION('center_axis',(0.,0.,1.));
#27665=DIRECTION('ref_axis',(1.,0.,0.));
#27666=DIRECTION('',(0.970134818690168,-0.242566348789345,0.));
#27667=DIRECTION('center_axis',(-0.242566348789345,-0.970134818690168,0.));
#27668=DIRECTION('ref_axis',(0.970134818690168,-0.242566348789345,0.));
#27669=DIRECTION('',(0.,0.,-1.));
#27670=DIRECTION('',(0.970134818690168,-0.242566348789345,0.));
#27671=DIRECTION('center_axis',(0.,0.,1.));
#27672=DIRECTION('ref_axis',(-0.707106781186548,0.707106781186548,0.));
#27673=DIRECTION('center_axis',(0.,0.,-1.));
#27674=DIRECTION('ref_axis',(1.,0.,0.));
#27675=DIRECTION('center_axis',(0.99985906712276,-0.0167882665098261,0.));
#27676=DIRECTION('ref_axis',(0.0167882665098261,0.99985906712276,0.));
#27677=DIRECTION('',(0.,0.,1.));
#27678=DIRECTION('',(0.0167882665098261,0.99985906712276,0.));
#27679=DIRECTION('',(0.,0.,1.));
#27680=DIRECTION('',(0.0167882665098261,0.99985906712276,0.));
#27681=DIRECTION('center_axis',(0.,0.,1.));
#27682=DIRECTION('ref_axis',(-0.5,0.866025403784439,0.));
#27683=DIRECTION('center_axis',(0.,0.,1.));
#27684=DIRECTION('ref_axis',(1.,0.,0.));
#27685=DIRECTION('',(0.874297485587433,-0.485390468278367,0.));
#27686=DIRECTION('center_axis',(-0.485390468278367,-0.874297485587433,0.));
#27687=DIRECTION('ref_axis',(0.874297485587433,-0.485390468278367,0.));
#27688=DIRECTION('',(0.,0.,-1.));
#27689=DIRECTION('',(0.874297485587433,-0.485390468278367,0.));
#27690=DIRECTION('center_axis',(0.,0.,1.));
#27691=DIRECTION('ref_axis',(-0.5,0.866025403784439,0.));
#27692=DIRECTION('center_axis',(0.,0.,-1.));
#27693=DIRECTION('ref_axis',(1.,0.,0.));
#27694=DIRECTION('center_axis',(0.961444572476169,-0.274998789190275,0.));
#27695=DIRECTION('ref_axis',(0.274998789190275,0.961444572476169,0.));
#27696=DIRECTION('',(0.,0.,1.));
#27697=DIRECTION('',(0.274998789190275,0.961444572476169,0.));
#27698=DIRECTION('',(0.,0.,1.));
#27699=DIRECTION('',(0.274998789190275,0.961444572476169,0.));
#27700=DIRECTION('center_axis',(0.,0.,1.));
#27701=DIRECTION('ref_axis',(-0.258819045102521,0.965925826289068,0.));
#27702=DIRECTION('center_axis',(0.,0.,1.));
#27703=DIRECTION('ref_axis',(1.,0.,0.));
#27704=DIRECTION('',(0.718878223686824,-0.695136029499894,0.));
#27705=DIRECTION('center_axis',(-0.695136029499894,-0.718878223686824,0.));
#27706=DIRECTION('ref_axis',(0.718878223686824,-0.695136029499894,0.));
#27707=DIRECTION('',(0.,0.,-1.));
#27708=DIRECTION('',(0.718878223686824,-0.695136029499894,0.));
#27709=DIRECTION('center_axis',(0.,0.,1.));
#27710=DIRECTION('ref_axis',(-0.258819045102521,0.965925826289068,0.));
#27711=DIRECTION('center_axis',(0.,0.,-1.));
#27712=DIRECTION('ref_axis',(1.,0.,0.));
#27713=DIRECTION('center_axis',(0.857509219077607,-0.514468598844393,0.));
#27714=DIRECTION('ref_axis',(0.514468598844393,0.857509219077607,0.));
#27715=DIRECTION('',(0.,0.,1.));
#27716=DIRECTION('',(0.514468598844393,0.857509219077607,0.));
#27717=DIRECTION('',(0.,0.,1.));
#27718=DIRECTION('',(0.514468598844393,0.857509219077607,0.));
#27719=DIRECTION('center_axis',(0.,0.,1.));
#27720=DIRECTION('ref_axis',(8.32667268468867E-17,1.,0.));
#27721=DIRECTION('center_axis',(0.,0.,1.));
#27722=DIRECTION('ref_axis',(1.,0.,0.));
#27723=DIRECTION('',(0.514468598844393,-0.857509219077607,0.));
#27724=DIRECTION('center_axis',(-0.857509219077607,-0.514468598844393,0.));
#27725=DIRECTION('ref_axis',(0.514468598844393,-0.857509219077607,0.));
#27726=DIRECTION('',(0.,0.,-1.));
#27727=DIRECTION('',(0.514468598844393,-0.857509219077607,0.));
#27728=DIRECTION('center_axis',(0.,0.,1.));
#27729=DIRECTION('ref_axis',(8.32667268468867E-17,1.,0.));
#27730=DIRECTION('center_axis',(0.,0.,-1.));
#27731=DIRECTION('ref_axis',(1.,0.,0.));
#27732=DIRECTION('center_axis',(0.695136029499894,-0.718878223686824,0.));
#27733=DIRECTION('ref_axis',(0.718878223686824,0.695136029499894,0.));
#27734=DIRECTION('',(0.,0.,1.));
#27735=DIRECTION('',(0.718878223686824,0.695136029499894,0.));
#27736=DIRECTION('',(0.,0.,1.));
#27737=DIRECTION('',(0.718878223686824,0.695136029499894,0.));
#27738=DIRECTION('center_axis',(0.,0.,1.));
#27739=DIRECTION('ref_axis',(0.258819045102521,0.965925826289068,0.));
#27740=DIRECTION('center_axis',(0.,0.,1.));
#27741=DIRECTION('ref_axis',(1.,0.,0.));
#27742=DIRECTION('',(0.274998789190274,-0.961444572476169,0.));
#27743=DIRECTION('center_axis',(-0.961444572476169,-0.274998789190274,0.));
#27744=DIRECTION('ref_axis',(0.274998789190274,-0.961444572476169,0.));
#27745=DIRECTION('',(0.,0.,-1.));
#27746=DIRECTION('',(0.274998789190274,-0.961444572476169,0.));
#27747=DIRECTION('center_axis',(0.,0.,1.));
#27748=DIRECTION('ref_axis',(0.258819045102521,0.965925826289068,0.));
#27749=DIRECTION('center_axis',(0.,0.,-1.));
#27750=DIRECTION('ref_axis',(1.,0.,0.));
#27751=DIRECTION('center_axis',(0.485390468278367,-0.874297485587433,0.));
#27752=DIRECTION('ref_axis',(0.874297485587433,0.485390468278367,0.));
#27753=DIRECTION('',(0.,0.,1.));
#27754=DIRECTION('',(0.874297485587433,0.485390468278367,0.));
#27755=DIRECTION('',(0.,0.,1.));
#27756=DIRECTION('',(0.874297485587433,0.485390468278367,0.));
#27757=DIRECTION('center_axis',(0.,0.,1.));
#27758=DIRECTION('ref_axis',(0.5,0.866025403784439,0.));
#27759=DIRECTION('center_axis',(0.,0.,1.));
#27760=DIRECTION('ref_axis',(1.,0.,0.));
#27761=DIRECTION('',(0.0167882665098258,-0.99985906712276,0.));
#27762=DIRECTION('center_axis',(-0.99985906712276,-0.0167882665098258,0.));
#27763=DIRECTION('ref_axis',(0.0167882665098258,-0.99985906712276,0.));
#27764=DIRECTION('',(0.,0.,-1.));
#27765=DIRECTION('',(0.0167882665098258,-0.99985906712276,0.));
#27766=DIRECTION('center_axis',(0.,0.,1.));
#27767=DIRECTION('ref_axis',(0.5,0.866025403784439,0.));
#27768=DIRECTION('center_axis',(0.,0.,-1.));
#27769=DIRECTION('ref_axis',(1.,0.,0.));
#27770=DIRECTION('center_axis',(0.242566348789345,-0.970134818690168,0.));
#27771=DIRECTION('ref_axis',(0.970134818690168,0.242566348789345,0.));
#27772=DIRECTION('',(0.,0.,1.));
#27773=DIRECTION('',(0.970134818690168,0.242566348789345,0.));
#27774=DIRECTION('',(0.,0.,1.));
#27775=DIRECTION('',(0.970134818690168,0.242566348789345,0.));
#27776=DIRECTION('center_axis',(0.,0.,1.));
#27777=DIRECTION('ref_axis',(0.707106781186547,0.707106781186548,0.));
#27778=DIRECTION('center_axis',(0.,0.,1.));
#27779=DIRECTION('ref_axis',(1.,0.,0.));
#27780=DIRECTION('',(-0.242566348789345,-0.970134818690168,0.));
#27781=DIRECTION('center_axis',(-0.970134818690168,0.242566348789345,0.));
#27782=DIRECTION('ref_axis',(-0.242566348789345,-0.970134818690168,0.));
#27783=DIRECTION('',(0.,0.,-1.));
#27784=DIRECTION('',(-0.242566348789345,-0.970134818690168,0.));
#27785=DIRECTION('center_axis',(0.,0.,1.));
#27786=DIRECTION('ref_axis',(0.707106781186547,0.707106781186548,0.));
#27787=DIRECTION('center_axis',(0.,0.,-1.));
#27788=DIRECTION('ref_axis',(1.,0.,0.));
#27789=DIRECTION('center_axis',(-0.0167882665098259,-0.99985906712276,0.));
#27790=DIRECTION('ref_axis',(0.99985906712276,-0.0167882665098259,0.));
#27791=DIRECTION('',(0.,0.,1.));
#27792=DIRECTION('',(0.99985906712276,-0.0167882665098259,0.));
#27793=DIRECTION('',(0.,0.,1.));
#27794=DIRECTION('',(0.99985906712276,-0.0167882665098259,0.));
#27795=DIRECTION('center_axis',(0.,0.,1.));
#27796=DIRECTION('ref_axis',(0.866025403784439,0.5,0.));
#27797=DIRECTION('center_axis',(0.,0.,1.));
#27798=DIRECTION('ref_axis',(1.,0.,0.));
#27799=DIRECTION('',(-0.485390468278367,-0.874297485587433,0.));
#27800=DIRECTION('center_axis',(-0.874297485587433,0.485390468278367,0.));
#27801=DIRECTION('ref_axis',(-0.485390468278367,-0.874297485587433,0.));
#27802=DIRECTION('',(0.,0.,-1.));
#27803=DIRECTION('',(-0.485390468278367,-0.874297485587433,0.));
#27804=DIRECTION('center_axis',(0.,0.,1.));
#27805=DIRECTION('ref_axis',(0.866025403784439,0.5,0.));
#27806=DIRECTION('center_axis',(0.,0.,-1.));
#27807=DIRECTION('ref_axis',(1.,0.,0.));
#27808=DIRECTION('center_axis',(-0.274998789190275,-0.961444572476169,0.));
#27809=DIRECTION('ref_axis',(0.961444572476169,-0.274998789190275,0.));
#27810=DIRECTION('',(0.,0.,1.));
#27811=DIRECTION('',(0.961444572476169,-0.274998789190275,0.));
#27812=DIRECTION('',(0.,0.,1.));
#27813=DIRECTION('',(0.961444572476169,-0.274998789190275,0.));
#27814=DIRECTION('center_axis',(0.,0.,1.));
#27815=DIRECTION('ref_axis',(0.965925826289068,0.258819045102521,0.));
#27816=DIRECTION('center_axis',(0.,0.,1.));
#27817=DIRECTION('ref_axis',(1.,0.,0.));
#27818=DIRECTION('',(-0.695136029499894,-0.718878223686824,0.));
#27819=DIRECTION('center_axis',(-0.718878223686824,0.695136029499894,0.));
#27820=DIRECTION('ref_axis',(-0.695136029499894,-0.718878223686824,0.));
#27821=DIRECTION('',(0.,0.,-1.));
#27822=DIRECTION('',(-0.695136029499894,-0.718878223686824,0.));
#27823=DIRECTION('center_axis',(0.,0.,1.));
#27824=DIRECTION('ref_axis',(0.965925826289068,0.258819045102521,0.));
#27825=DIRECTION('center_axis',(0.,0.,-1.));
#27826=DIRECTION('ref_axis',(1.,0.,0.));
#27827=DIRECTION('center_axis',(-0.514468598844393,-0.857509219077607,0.));
#27828=DIRECTION('ref_axis',(0.857509219077607,-0.514468598844393,0.));
#27829=DIRECTION('',(0.,0.,1.));
#27830=DIRECTION('',(0.857509219077607,-0.514468598844393,0.));
#27831=DIRECTION('',(0.,0.,1.));
#27832=DIRECTION('',(0.857509219077607,-0.514468598844393,0.));
#27833=DIRECTION('center_axis',(0.,0.,1.));
#27834=DIRECTION('ref_axis',(1.,0.,0.));
#27835=DIRECTION('center_axis',(0.,0.,1.));
#27836=DIRECTION('ref_axis',(1.,0.,0.));
#27837=DIRECTION('',(-0.857509219077607,-0.514468598844393,0.));
#27838=DIRECTION('center_axis',(-0.514468598844393,0.857509219077607,0.));
#27839=DIRECTION('ref_axis',(-0.857509219077607,-0.514468598844393,0.));
#27840=DIRECTION('',(0.,0.,-1.));
#27841=DIRECTION('',(-0.857509219077607,-0.514468598844393,0.));
#27842=DIRECTION('center_axis',(0.,0.,1.));
#27843=DIRECTION('ref_axis',(1.,0.,0.));
#27844=DIRECTION('center_axis',(0.,0.,-1.));
#27845=DIRECTION('ref_axis',(1.,0.,0.));
#27846=DIRECTION('center_axis',(0.,0.,1.));
#27847=DIRECTION('ref_axis',(1.,0.,0.));
#27848=DIRECTION('center_axis',(0.,0.,1.));
#27849=DIRECTION('ref_axis',(1.,0.,0.));
#27850=DIRECTION('',(0.,0.,-1.));
#27851=DIRECTION('center_axis',(0.,0.,-1.));
#27852=DIRECTION('ref_axis',(1.,0.,0.));
#27853=DIRECTION('center_axis',(0.,0.,-1.));
#27854=DIRECTION('ref_axis',(1.,0.,0.));
#27855=DIRECTION('center_axis',(0.,0.,1.));
#27856=DIRECTION('ref_axis',(1.,0.,0.));
#27857=DIRECTION('',(-0.600000000000002,-7.34788079488414E-17,-0.799999999999999));
#27858=DIRECTION('center_axis',(0.,0.,1.));
#27859=DIRECTION('ref_axis',(1.,0.,0.));
#27860=DIRECTION('center_axis',(0.,0.,-1.));
#27861=DIRECTION('ref_axis',(-1.,0.,0.));
#27862=DIRECTION('center_axis',(0.,0.,1.));
#27863=DIRECTION('ref_axis',(1.,0.,0.));
#27864=DIRECTION('center_axis',(0.,0.,1.));
#27865=DIRECTION('ref_axis',(1.,0.,0.));
#27866=DIRECTION('',(0.,0.,1.));
#27867=DIRECTION('center_axis',(0.,0.,-1.));
#27868=DIRECTION('ref_axis',(1.,0.,0.));
#27869=DIRECTION('center_axis',(0.,0.,1.));
#27870=DIRECTION('ref_axis',(1.,0.,0.));
#27871=DIRECTION('center_axis',(0.,0.,1.));
#27872=DIRECTION('ref_axis',(1.,0.,0.));
#27873=DIRECTION('',(0.,0.,-1.));
#27874=DIRECTION('',(0.,0.,-1.));
#27875=DIRECTION('center_axis',(0.,0.,-1.));
#27876=DIRECTION('ref_axis',(1.,0.,0.));
#27877=DIRECTION('center_axis',(0.,0.,-1.));
#27878=DIRECTION('ref_axis',(-1.,0.,0.));
#27879=DIRECTION('center_axis',(0.,0.,1.));
#27880=DIRECTION('ref_axis',(1.,0.,0.));
#27881=DIRECTION('center_axis',(0.,0.,1.));
#27882=DIRECTION('ref_axis',(1.,0.,0.));
#27883=DIRECTION('center_axis',(0.,0.,1.));
#27884=DIRECTION('ref_axis',(1.,0.,0.));
#27885=DIRECTION('',(0.,0.,-1.));
#27886=DIRECTION('center_axis',(0.,0.,-1.));
#27887=DIRECTION('ref_axis',(1.,0.,0.));
#27888=DIRECTION('center_axis',(0.,0.,1.));
#27889=DIRECTION('ref_axis',(1.,0.,0.));
#27890=DIRECTION('',(-0.70710678118655,-8.65956056235496E-17,-0.707106781186545));
#27891=DIRECTION('center_axis',(0.,0.,1.));
#27892=DIRECTION('ref_axis',(1.,0.,0.));
#27893=DIRECTION('center_axis',(-3.49629579342466E-16,-1.,0.));
#27894=DIRECTION('ref_axis',(1.,-3.49629579342466E-16,0.));
#27895=DIRECTION('',(-1.,3.49629579342466E-16,0.));
#27896=DIRECTION('',(0.,0.,1.));
#27897=DIRECTION('',(1.,-3.49629579342466E-16,0.));
#27898=DIRECTION('',(0.,0.,1.));
#27899=DIRECTION('center_axis',(-0.866025403784439,-0.5,0.));
#27900=DIRECTION('ref_axis',(0.5,-0.866025403784439,0.));
#27901=DIRECTION('',(-0.5,0.866025403784439,0.));
#27902=DIRECTION('',(0.5,-0.866025403784439,0.));
#27903=DIRECTION('',(0.,0.,1.));
#27904=DIRECTION('center_axis',(-0.866025403784439,0.5,0.));
#27905=DIRECTION('ref_axis',(-0.5,-0.866025403784439,0.));
#27906=DIRECTION('',(0.5,0.866025403784439,0.));
#27907=DIRECTION('',(-0.5,-0.866025403784439,0.));
#27908=DIRECTION('',(0.,0.,1.));
#27909=DIRECTION('center_axis',(1.74814789671233E-16,1.,0.));
#27910=DIRECTION('ref_axis',(-1.,1.74814789671233E-16,0.));
#27911=DIRECTION('',(1.,-1.74814789671233E-16,0.));
#27912=DIRECTION('',(-1.,1.74814789671233E-16,0.));
#27913=DIRECTION('',(0.,0.,1.));
#27914=DIRECTION('center_axis',(0.866025403784439,0.5,0.));
#27915=DIRECTION('ref_axis',(-0.5,0.866025403784439,0.));
#27916=DIRECTION('',(0.5,-0.866025403784439,0.));
#27917=DIRECTION('',(-0.5,0.866025403784439,0.));
#27918=DIRECTION('',(0.,0.,1.));
#27919=DIRECTION('center_axis',(0.866025403784439,-0.5,0.));
#27920=DIRECTION('ref_axis',(0.5,0.866025403784439,0.));
#27921=DIRECTION('',(-0.5,-0.866025403784439,0.));
#27922=DIRECTION('',(0.5,0.866025403784439,0.));
#27923=DIRECTION('center_axis',(0.,0.,1.));
#27924=DIRECTION('ref_axis',(1.,0.,0.));
#27925=DIRECTION('center_axis',(0.,0.,1.));
#27926=DIRECTION('ref_axis',(1.,0.,0.));
#27927=DIRECTION('',(0.,-1.,0.));
#27928=DIRECTION('',(-1.,0.,0.));
#27929=DIRECTION('',(0.,1.,0.));
#27930=DIRECTION('',(1.,0.,0.));
#27931=DIRECTION('center_axis',(0.,0.,-1.));
#27932=DIRECTION('ref_axis',(1.,0.,0.));
#27933=DIRECTION('center_axis',(0.,1.,0.));
#27934=DIRECTION('ref_axis',(-1.,0.,0.));
#27935=DIRECTION('',(0.,0.,1.));
#27936=DIRECTION('',(-1.,0.,0.));
#27937=DIRECTION('',(0.,0.,1.));
#27938=DIRECTION('center_axis',(1.,0.,0.));
#27939=DIRECTION('ref_axis',(0.,1.,0.));
#27940=DIRECTION('',(0.,1.,0.));
#27941=DIRECTION('',(0.,0.,1.));
#27942=DIRECTION('center_axis',(0.,-1.,0.));
#27943=DIRECTION('ref_axis',(1.,0.,0.));
#27944=DIRECTION('',(1.,0.,0.));
#27945=DIRECTION('',(0.,0.,1.));
#27946=DIRECTION('center_axis',(-1.,0.,0.));
#27947=DIRECTION('ref_axis',(0.,-1.,0.));
#27948=DIRECTION('',(0.,-1.,0.));
#27949=DIRECTION('center_axis',(0.,0.,1.));
#27950=DIRECTION('ref_axis',(1.,0.,0.));
#27951=DIRECTION('center_axis',(0.,0.,-1.));
#27952=DIRECTION('ref_axis',(-1.,0.,0.));
#27953=DIRECTION('center_axis',(0.,0.,1.));
#27954=DIRECTION('ref_axis',(1.,0.,0.));
#27955=DIRECTION('center_axis',(0.,0.,1.));
#27956=DIRECTION('ref_axis',(1.,0.,0.));
#27957=DIRECTION('',(0.707106781186548,8.65956056235493E-17,-0.707106781186548));
#27958=DIRECTION('center_axis',(0.,0.,1.));
#27959=DIRECTION('ref_axis',(1.,0.,0.));
#33233=CARTESIAN_POINT('',(0.,0.,0.));
#33234=CARTESIAN_POINT('Origin',(0.,0.,-0.48));
#33235=CARTESIAN_POINT('',(-0.395253163807729,0.000335471986130265,-0.715584015536924));
#33236=CARTESIAN_POINT('',(-0.395255438336,0.000332125708880706,-0.726115984463077));
#33237=CARTESIAN_POINT('',(-0.3954,-4.84225344382863E-17,-0.48));
#33238=CARTESIAN_POINT('',(-0.395861479162046,-0.000213366483867161,-0.790584015536923));
#33239=CARTESIAN_POINT('Ctrl Pts',(-0.395253163807729,0.000335471986130265,
-0.715584015536924));
#33240=CARTESIAN_POINT('Ctrl Pts',(-0.395551653151419,0.0357534542470482,
-0.716652535192449));
#33241=CARTESIAN_POINT('Ctrl Pts',(-0.391174119565203,0.0710989968386545,
-0.717721054847974));
#33242=CARTESIAN_POINT('Ctrl Pts',(-0.381823957673672,0.105076140411834,
-0.718789574503499));
#33243=CARTESIAN_POINT('Ctrl Pts',(-0.347453343346403,0.22997400969405,
-0.722717386386032));
#33244=CARTESIAN_POINT('Ctrl Pts',(-0.2458899929036,0.336381360783369,-0.726645198268564));
#33245=CARTESIAN_POINT('Ctrl Pts',(-0.122725269859081,0.376524449371095,
-0.730573010151097));
#33246=CARTESIAN_POINT('Ctrl Pts',(0.000439453185439045,0.416667537958822,
-0.73450082203363));
#33247=CARTESIAN_POINT('Ctrl Pts',(0.145205548831676,0.390546364044954,
-0.738428633916163));
#33248=CARTESIAN_POINT('Ctrl Pts',(0.246571894502321,0.309893277568692,
-0.742356445798696));
#33249=CARTESIAN_POINT('Ctrl Pts',(0.347938240172965,0.229240191092431,
-0.746284257681229));
#33250=CARTESIAN_POINT('Ctrl Pts',(0.405904835868018,0.0940551920537777,
-0.750212069563761));
#33251=CARTESIAN_POINT('Ctrl Pts',(0.394465702582075,-0.0349816075370925,
-0.754139881446293));
#33252=CARTESIAN_POINT('Ctrl Pts',(0.383026569296131,-0.164018407127964,
-0.758067693328826));
#33253=CARTESIAN_POINT('Ctrl Pts',(0.302181707029189,-0.286907007271051,
-0.76199550521136));
#33254=CARTESIAN_POINT('Ctrl Pts',(0.188191962309989,-0.348457576111146,
-0.765923317093893));
#33255=CARTESIAN_POINT('Ctrl Pts',(0.0742022175907893,-0.41000814495124,
-0.769851128976425));
#33256=CARTESIAN_POINT('Ctrl Pts',(-0.0729324095806676,-0.410220682488342,
-0.773778940858958));
#33257=CARTESIAN_POINT('Ctrl Pts',(-0.18709178097685,-0.349037578722476,
-0.77770675274149));
#33258=CARTESIAN_POINT('Ctrl Pts',(-0.301251152373033,-0.287854474956611,
-0.781634564624023));
#33259=CARTESIAN_POINT('Ctrl Pts',(-0.382435267993942,-0.165275729887777,
-0.785562376506555));
#33260=CARTESIAN_POINT('Ctrl Pts',(-0.394322160558364,-0.0362597276125358,
-0.789490188389088));
#33261=CARTESIAN_POINT('Ctrl Pts',(-0.395425591355561,-0.0242834916475591,
-0.789854797438367));
#33262=CARTESIAN_POINT('Ctrl Pts',(-0.395931891509389,-0.0122517861649356,
-0.790219406487645));
#33263=CARTESIAN_POINT('Ctrl Pts',(-0.395861479162046,-0.000213366483867161,
-0.790584015536923));
#33264=CARTESIAN_POINT('',(-0.3954,-4.84225344382863E-17,-0.9646));
#33265=CARTESIAN_POINT('',(-0.3954,-4.84225344382863E-17,-0.48));
#33266=CARTESIAN_POINT('Origin',(0.,0.,-0.9646));
#33267=CARTESIAN_POINT('',(-0.278857777366742,0.281064285032673,-0.800000000000001));
#33268=CARTESIAN_POINT('Ctrl Pts',(-0.395861479162046,-0.000213366483867161,
-0.790584015536923));
#33269=CARTESIAN_POINT('Ctrl Pts',(-0.39525534905282,0.10341687610184,-0.793722677024616));
#33270=CARTESIAN_POINT('Ctrl Pts',(-0.351913261714371,0.207544658964529,
-0.796861338512308));
#33271=CARTESIAN_POINT('Ctrl Pts',(-0.278859905177388,0.28106907114812,
-0.800000000000001));
#33272=CARTESIAN_POINT('',(-0.393673192958032,-0.0369131026361662,-0.8));
#33273=CARTESIAN_POINT('Origin',(0.,0.,-0.8));
#33274=CARTESIAN_POINT('Ctrl Pts',(-0.393673192958032,-0.0369131026361654,
-0.8));
#33275=CARTESIAN_POINT('Ctrl Pts',(-0.381526729866673,-0.166453470874879,
-0.796072188117467));
#33276=CARTESIAN_POINT('Ctrl Pts',(-0.300626129406055,-0.288465681742495,
-0.792144376234934));
#33277=CARTESIAN_POINT('Ctrl Pts',(-0.186505338687462,-0.349319299154459,
-0.788216564352402));
#33278=CARTESIAN_POINT('Ctrl Pts',(-0.0723845479688678,-0.410172916566423,
-0.784288752469869));
#33279=CARTESIAN_POINT('Ctrl Pts',(0.0749564330077028,-0.409867940522735,
-0.780360940587336));
#33280=CARTESIAN_POINT('Ctrl Pts',(0.188884746658086,-0.348150998874613,
-0.776433128704804));
#33281=CARTESIAN_POINT('Ctrl Pts',(0.302813060308468,-0.286434057226491,
-0.772505316822271));
#33282=CARTESIAN_POINT('Ctrl Pts',(0.383328706632664,-0.163305149973936,
-0.768577504939738));
#33283=CARTESIAN_POINT('Ctrl Pts',(0.394503823024529,-0.0342255654622517,
-0.764649693057205));
#33284=CARTESIAN_POINT('Ctrl Pts',(0.405678939416394,0.0948540190494324,
-0.760721881174672));
#33285=CARTESIAN_POINT('Ctrl Pts',(0.347513525875929,0.229884280820245,
-0.756794069292139));
#33286=CARTESIAN_POINT('Ctrl Pts',(0.246010089847033,0.310337863189681,
-0.752866257409607));
#33287=CARTESIAN_POINT('Ctrl Pts',(0.144506653818137,0.390791445559116,
-0.748938445527074));
#33288=CARTESIAN_POINT('Ctrl Pts',(-0.000334804699189922,0.416668348527174,
-0.745010633644541));
#33289=CARTESIAN_POINT('Ctrl Pts',(-0.12343126021814,0.376302547448928,
-0.741082821762008));
#33290=CARTESIAN_POINT('Ctrl Pts',(-0.24652771573709,0.335936746370681,
-0.737155009879476));
#33291=CARTESIAN_POINT('Ctrl Pts',(-0.347879168257662,0.22932824124613,
-0.733227197996943));
#33292=CARTESIAN_POINT('Ctrl Pts',(-0.382014496854013,0.104363742597582,
-0.72929938611441));
#33293=CARTESIAN_POINT('Ctrl Pts',(-0.391236464425464,0.070603453726573,
-0.728238252230632));
#33294=CARTESIAN_POINT('Ctrl Pts',(-0.395552602268709,0.035503436030642,
-0.727177118346855));
#33295=CARTESIAN_POINT('Ctrl Pts',(-0.395255438336,0.000332125708880706,
-0.726115984463077));
#33296=CARTESIAN_POINT('Origin',(0.,0.,-0.48));
#33297=CARTESIAN_POINT('',(-0.394965714787616,-0.000250953455007918,-0.640584015536923));
#33298=CARTESIAN_POINT('',(-0.394960834327206,-0.000248313920574979,-0.651115984463077));
#33299=CARTESIAN_POINT('',(-0.3954,-4.84225344382863E-17,-0.48));
#33300=CARTESIAN_POINT('Ctrl Pts',(-0.394965714787616,-0.000250953455007918,
-0.640584015536923));
#33301=CARTESIAN_POINT('Ctrl Pts',(-0.394471046036972,0.0828241788087287,
-0.643085663897252));
#33302=CARTESIAN_POINT('Ctrl Pts',(-0.368812762630574,0.166178887533591,
-0.64558731225758));
#33303=CARTESIAN_POINT('Ctrl Pts',(-0.320289765331127,0.232906929873211,
-0.648088960617908));
#33304=CARTESIAN_POINT('Ctrl Pts',(-0.244104315612744,0.337675930087654,
-0.652016772500441));
#33305=CARTESIAN_POINT('Ctrl Pts',(-0.111553205064048,0.401457186366483,
-0.655944584382975));
#33306=CARTESIAN_POINT('Ctrl Pts',(0.0178556785537009,0.395616446478012,
-0.659872396265507));
#33307=CARTESIAN_POINT('Ctrl Pts',(0.14726456217145,0.389775706589541,-0.66380020814804));
#33308=CARTESIAN_POINT('Ctrl Pts',(0.27353121885825,0.314312970533769,-0.667728020030573));
#33309=CARTESIAN_POINT('Ctrl Pts',(0.339968835940365,0.203106870469053,
-0.671655831913105));
#33310=CARTESIAN_POINT('Ctrl Pts',(0.40640645302248,0.091900770404338,-0.675583643795638));
#33311=CARTESIAN_POINT('Ctrl Pts',(0.413015030499909,-0.0550486936693204,
-0.679511455678171));
#33312=CARTESIAN_POINT('Ctrl Pts',(0.356828054007659,-0.171769696291924,
-0.683439267560704));
#33313=CARTESIAN_POINT('Ctrl Pts',(0.300641077515409,-0.288490698914528,
-0.687367079443237));
#33314=CARTESIAN_POINT('Ctrl Pts',(0.181658547053481,-0.374983240086078,
-0.691294891325769));
#33315=CARTESIAN_POINT('Ctrl Pts',(0.0532962243198568,-0.392416631099017,
-0.695222703208302));
#33316=CARTESIAN_POINT('Ctrl Pts',(-0.0750660984137688,-0.409850022111956,
-0.699150515090834));
#33317=CARTESIAN_POINT('Ctrl Pts',(-0.212808213419091,-0.358224262966283,
-0.703078326973367));
#33318=CARTESIAN_POINT('Ctrl Pts',(-0.298090331815884,-0.260717189655889,
-0.7070061388559));
#33319=CARTESIAN_POINT('Ctrl Pts',(-0.360172352423616,-0.189735883744952,
-0.709865431082908));
#33320=CARTESIAN_POINT('Ctrl Pts',(-0.394454424864704,-0.0944408485534943,
-0.712724723309916));
#33321=CARTESIAN_POINT('Ctrl Pts',(-0.395253163807729,0.000335471986130265,
-0.715584015536924));
#33322=CARTESIAN_POINT('Ctrl Pts',(-0.395255438336,0.000332125708880706,
-0.726115984463077));
#33323=CARTESIAN_POINT('Ctrl Pts',(-0.394452643023416,-0.0946839915107613,
-0.723249306464322));
#33324=CARTESIAN_POINT('Ctrl Pts',(-0.35998091681832,-0.190220418610138,
-0.720382628465567));
#33325=CARTESIAN_POINT('Ctrl Pts',(-0.297607838874384,-0.261268242344166,
-0.717515950466812));
#33326=CARTESIAN_POINT('Ctrl Pts',(-0.212146647626277,-0.358615236464823,
-0.713588138584279));
#33327=CARTESIAN_POINT('Ctrl Pts',(-0.0743050604579336,-0.409988732533595,
-0.709660326701746));
#33328=CARTESIAN_POINT('Ctrl Pts',(0.054025596928822,-0.392317937929058,
-0.705732514819213));
#33329=CARTESIAN_POINT('Ctrl Pts',(0.182356254315577,-0.37464714332452,
-0.70180470293668));
#33330=CARTESIAN_POINT('Ctrl Pts',(0.301175981920744,-0.287932058046674,
-0.697876891054148));
#33331=CARTESIAN_POINT('Ctrl Pts',(0.357145708980789,-0.171106530935462,
-0.693949079171615));
#33332=CARTESIAN_POINT('Ctrl Pts',(0.413115436040835,-0.0542810038242487,
-0.690021267289082));
#33333=CARTESIAN_POINT('Ctrl Pts',(0.406235162555757,0.0926549651203302,
-0.686093455406549));
#33334=CARTESIAN_POINT('Ctrl Pts',(0.339591493502025,0.20373731066395,-0.682165643524016));
#33335=CARTESIAN_POINT('Ctrl Pts',(0.272947824448293,0.314819656207569,
-0.678237831641484));
#33336=CARTESIAN_POINT('Ctrl Pts',(0.146540759825906,0.39004837835023,-0.674310019758951));
#33337=CARTESIAN_POINT('Ctrl Pts',(0.0171211347676443,0.395649013122802,
-0.670382207876419));
#33338=CARTESIAN_POINT('Ctrl Pts',(-0.112298490290618,0.401249647895373,
-0.666454395993886));
#33339=CARTESIAN_POINT('Ctrl Pts',(-0.244730675784755,0.337222195297856,
-0.662526584111353));
#33340=CARTESIAN_POINT('Ctrl Pts',(-0.320721441453192,0.232311902261895,
-0.65859877222882));
#33341=CARTESIAN_POINT('Ctrl Pts',(-0.368977551866046,0.165691140651501,
-0.656104509640239));
#33342=CARTESIAN_POINT('Ctrl Pts',(-0.394473208494698,0.0825840467829949,
-0.653610247051658));
#33343=CARTESIAN_POINT('Ctrl Pts',(-0.394960834327206,-0.000248313920574979,
-0.651115984463077));
#33344=CARTESIAN_POINT('Origin',(0.,0.,-0.48));
#33345=CARTESIAN_POINT('',(-0.39601914064734,4.10564873420969E-6,-0.565584015536924));
#33346=CARTESIAN_POINT('',(-0.396019157300021,-2.47054920110875E-7,-0.576115984463077));
#33347=CARTESIAN_POINT('',(-0.3954,-4.84225344382863E-17,-0.48));
#33348=CARTESIAN_POINT('Ctrl Pts',(-0.396019115773222,4.10548378882781E-6,
-0.565584015536924));
#33349=CARTESIAN_POINT('Ctrl Pts',(-0.396039459492,0.129774468910247,-0.569518792602056));
#33350=CARTESIAN_POINT('Ctrl Pts',(-0.326064226544098,0.259525796747945,
-0.573453569667187));
#33351=CARTESIAN_POINT('Ctrl Pts',(-0.217650027597511,0.330846869196683,
-0.577388346732319));
#33352=CARTESIAN_POINT('Ctrl Pts',(-0.109427739064012,0.402041691978786,
-0.581316158614852));
#33353=CARTESIAN_POINT('Ctrl Pts',(0.0370973536411718,0.415012938357412,
-0.585243970497384));
#33354=CARTESIAN_POINT('Ctrl Pts',(0.156143733414188,0.363937247625334,
-0.589171782379917));
#33355=CARTESIAN_POINT('Ctrl Pts',(0.275190113187202,0.312861556893256,
-0.59309959426245));
#33356=CARTESIAN_POINT('Ctrl Pts',(0.366757780028048,0.197738929050475,
-0.597027406144982));
#33357=CARTESIAN_POINT('Ctrl Pts',(0.389738001674511,0.0702529463705541,
-0.600955218027515));
#33358=CARTESIAN_POINT('Ctrl Pts',(0.412718223320974,-0.0572330363093691,
-0.604883029910048));
#33359=CARTESIAN_POINT('Ctrl Pts',(0.367110999773051,-0.197082373826433,
-0.608810841792581));
#33360=CARTESIAN_POINT('Ctrl Pts',(0.27339141480735,-0.286510589711546,
-0.612738653675114));
#33361=CARTESIAN_POINT('Ctrl Pts',(0.179671829841651,-0.375938805596657,
-0.616666465557647));
#33362=CARTESIAN_POINT('Ctrl Pts',(0.0378398834581742,-0.414945899849817,
-0.620594277440179));
#33363=CARTESIAN_POINT('Ctrl Pts',(-0.0884298780502877,-0.386019874399458,
-0.624522089322712));
#33364=CARTESIAN_POINT('Ctrl Pts',(-0.21469963955875,-0.357093848949099,
-0.628449901205245));
#33365=CARTESIAN_POINT('Ctrl Pts',(-0.325407216192197,-0.260234703795221,
-0.632377713087778));
#33366=CARTESIAN_POINT('Ctrl Pts',(-0.370851110064887,-0.138926759143254,
-0.63630552497031));
#33367=CARTESIAN_POINT('Ctrl Pts',(-0.387351499005705,-0.0948806156948923,
-0.637731688492515));
#33368=CARTESIAN_POINT('Ctrl Pts',(-0.395247720260061,-0.0476112160385504,
-0.639157852014719));
#33369=CARTESIAN_POINT('Ctrl Pts',(-0.394965714787616,-0.000250953455007918,
-0.640584015536923));
#33370=CARTESIAN_POINT('Ctrl Pts',(-0.394960834327206,-0.000248313920574979,
-0.651115984463077));
#33371=CARTESIAN_POINT('Ctrl Pts',(-0.395241091775281,-0.0478552791000078,
-0.649682435169125));
#33372=CARTESIAN_POINT('Ctrl Pts',(-0.387260581472885,-0.0953714931568358,
-0.648248885875173));
#33373=CARTESIAN_POINT('Ctrl Pts',(-0.37059260016416,-0.139614862151827,
-0.646815336581222));
#33374=CARTESIAN_POINT('Ctrl Pts',(-0.324923647363953,-0.260838200055182,
-0.642887524698689));
#33375=CARTESIAN_POINT('Ctrl Pts',(-0.214036395920803,-0.357491742387486,
-0.638959712816156));
#33376=CARTESIAN_POINT('Ctrl Pts',(-0.0877131492638707,-0.386183345199099,
-0.635031900933623));
#33377=CARTESIAN_POINT('Ctrl Pts',(0.0386100973930622,-0.414874948010711,
-0.63110408905109));
#33378=CARTESIAN_POINT('Ctrl Pts',(0.180369339263778,-0.375604611301632,
-0.627176277168558));
#33379=CARTESIAN_POINT('Ctrl Pts',(0.273922744458712,-0.286002581116925,
-0.623248465286025));
#33380=CARTESIAN_POINT('Ctrl Pts',(0.367476149653647,-0.196400550932217,
-0.619320653403493));
#33381=CARTESIAN_POINT('Ctrl Pts',(0.412823718172801,-0.0564668272718801,
-0.615392841520959));
#33382=CARTESIAN_POINT('Ctrl Pts',(0.389606897901208,0.070976263805676,
-0.611465029638427));
#33383=CARTESIAN_POINT('Ctrl Pts',(0.366390077629615,0.198419354883232,
-0.607537217755894));
#33384=CARTESIAN_POINT('Ctrl Pts',(0.274608868567275,0.313371813378008,
-0.603609405873361));
#33385=CARTESIAN_POINT('Ctrl Pts',(0.155467891744039,0.364226435131106,
-0.599681593990828));
#33386=CARTESIAN_POINT('Ctrl Pts',(0.0363269149208032,0.415081056884205,
-0.595753782108295));
#33387=CARTESIAN_POINT('Ctrl Pts',(-0.110173829663326,0.401837841895627,
-0.591825970225762));
#33388=CARTESIAN_POINT('Ctrl Pts',(-0.21826376648398,0.330442259074028,
-0.58789815834323));
#33389=CARTESIAN_POINT('Ctrl Pts',(-0.326342129060288,0.259054321274205,
-0.583970767049845));
#33390=CARTESIAN_POINT('Ctrl Pts',(-0.396017909472745,0.129526468857604,
-0.580043375756461));
#33391=CARTESIAN_POINT('Ctrl Pts',(-0.396019142095646,-2.47048853291312E-7,
-0.576115984463077));
#33392=CARTESIAN_POINT('Origin',(0.,0.,-0.48));
#33393=CARTESIAN_POINT('',(-0.394956676078496,0.000245896443633459,-0.490584015536923));
#33394=CARTESIAN_POINT('',(-0.394961414894976,0.000248589851300403,-0.501115984463076));
#33395=CARTESIAN_POINT('',(-0.3954,-4.84225344382863E-17,-0.48));
#33396=CARTESIAN_POINT('Ctrl Pts',(-0.394956676078496,0.000245896443633459,
-0.490584015536923));
#33397=CARTESIAN_POINT('Ctrl Pts',(-0.395235276024708,0.0480715230603383,
-0.492024109424326));
#33398=CARTESIAN_POINT('Ctrl Pts',(-0.387179611885601,0.0958065206795767,
-0.493464203311728));
#33399=CARTESIAN_POINT('Ctrl Pts',(-0.370362436155785,0.140224290031149,
-0.49490429719913));
#33400=CARTESIAN_POINT('Ctrl Pts',(-0.324494105458702,0.261372392790905,
-0.498832109081663));
#33401=CARTESIAN_POINT('Ctrl Pts',(-0.213448111654675,0.357843339760786,
-0.502759920964196));
#33402=CARTESIAN_POINT('Ctrl Pts',(-0.0870778555314957,0.386327105829989,
-0.506687732846729));
#33403=CARTESIAN_POINT('Ctrl Pts',(0.0392924005916832,0.414810871899191,
-0.510615544729262));
#33404=CARTESIAN_POINT('Ctrl Pts',(0.180986919034015,0.375307457067717,
-0.514543356611794));
#33405=CARTESIAN_POINT('Ctrl Pts',(0.274392836624718,0.285551671039299,
-0.518471168494327));
#33406=CARTESIAN_POINT('Ctrl Pts',(0.367798754215423,0.19579588501088,-0.52239898037686));
#33407=CARTESIAN_POINT('Ctrl Pts',(0.412916070954497,0.0557877277855151,
-0.526326792259393));
#33408=CARTESIAN_POINT('Ctrl Pts',(0.389489651066459,-0.0716170186429137,
-0.530254604141926));
#33409=CARTESIAN_POINT('Ctrl Pts',(0.366063231178422,-0.19902176507134,
-0.534182416024458));
#33410=CARTESIAN_POINT('Ctrl Pts',(0.274093074663277,-0.31382310070283,
-0.538110227906991));
#33411=CARTESIAN_POINT('Ctrl Pts',(0.154868605220906,-0.36448168775808,
-0.542038039789524));
#33412=CARTESIAN_POINT('Ctrl Pts',(0.0356441357785338,-0.415140274813329,
-0.545965851672056));
#33413=CARTESIAN_POINT('Ctrl Pts',(-0.110834646591064,-0.401656113292336,
-0.549893663554589));
#33414=CARTESIAN_POINT('Ctrl Pts',(-0.218807013758192,-0.330082832562713,
-0.553821475437122));
#33415=CARTESIAN_POINT('Ctrl Pts',(-0.326587913697395,-0.258636472618604,
-0.557742322137056));
#33416=CARTESIAN_POINT('Ctrl Pts',(-0.395998844077695,-0.129306829485993,
-0.56166316883699));
#33417=CARTESIAN_POINT('Ctrl Pts',(-0.396019115773222,4.10548378882781E-6,
-0.565584015536924));
#33418=CARTESIAN_POINT('Ctrl Pts',(-0.396019142095646,-2.47048853291312E-7,
-0.576115984463077));
#33419=CARTESIAN_POINT('Ctrl Pts',(-0.396020374982553,-0.129554705304902,
-0.572187751991396));
#33420=CARTESIAN_POINT('Ctrl Pts',(-0.326310510095658,-0.259108025856776,
-0.568259519519714));
#33421=CARTESIAN_POINT('Ctrl Pts',(-0.218193903826923,-0.330488397181274,
-0.564331287048033));
#33422=CARTESIAN_POINT('Ctrl Pts',(-0.11008887341875,-0.401861125931206,
-0.5604034751655));
#33423=CARTESIAN_POINT('Ctrl Pts',(0.0364146738056535,-0.415073361743801,
-0.556475663282968));
#33424=CARTESIAN_POINT('Ctrl Pts',(0.155544893218128,-0.364193555966734,
-0.552547851400435));
#33425=CARTESIAN_POINT('Ctrl Pts',(0.274675112630603,-0.313313750189668,
-0.548620039517903));
#33426=CARTESIAN_POINT('Ctrl Pts',(0.366432004231147,-0.198341902822938,
-0.544692227635369));
#33427=CARTESIAN_POINT('Ctrl Pts',(0.389621887462813,-0.0708939010958812,
-0.540764415752836));
#33428=CARTESIAN_POINT('Ctrl Pts',(0.412811770694479,0.056554100631176,
-0.536836603870304));
#33429=CARTESIAN_POINT('Ctrl Pts',(0.367434645557268,0.196478256718561,
-0.532908791987771));
#33430=CARTESIAN_POINT('Ctrl Pts',(0.273862287592234,0.286060496577444,
-0.528980980105239));
#33431=CARTESIAN_POINT('Ctrl Pts',(0.1802899296272,0.375642736436327,-0.525053168222706));
#33432=CARTESIAN_POINT('Ctrl Pts',(0.0385223388343421,0.414883060066708,
-0.521125356340173));
#33433=CARTESIAN_POINT('Ctrl Pts',(-0.0877948164623846,0.386164771103267,
-0.51719754445764));
#33434=CARTESIAN_POINT('Ctrl Pts',(-0.214111971759111,0.357446482139827,
-0.513269732575107));
#33435=CARTESIAN_POINT('Ctrl Pts',(-0.324978691559707,0.260769580582567,
-0.509341920692574));
#33436=CARTESIAN_POINT('Ctrl Pts',(-0.370622058898363,0.139536553455912,
-0.505414108810041));
#33437=CARTESIAN_POINT('Ctrl Pts',(-0.387270927216809,0.0953156113527008,
-0.503981400694386));
#33438=CARTESIAN_POINT('Ctrl Pts',(-0.395241844399756,0.0478274827323181,
-0.502548692578731));
#33439=CARTESIAN_POINT('Ctrl Pts',(-0.394961414894976,0.000248589851300403,
-0.501115984463076));
#33440=CARTESIAN_POINT('Origin',(0.,0.,-0.48));
#33441=CARTESIAN_POINT('',(-0.395266933374857,-0.000337325613274597,-0.415584015536924));
#33442=CARTESIAN_POINT('',(-0.395260053944926,-0.00033663270935099,-0.426115984463076));
#33443=CARTESIAN_POINT('',(-0.3954,-4.84225344382863E-17,-0.48));
#33444=CARTESIAN_POINT('Ctrl Pts',(-0.395266933374857,-0.000337325613274597,
-0.415584015536924));
#33445=CARTESIAN_POINT('Ctrl Pts',(-0.394458698757483,0.0948929263788777,
-0.418457238129129));
#33446=CARTESIAN_POINT('Ctrl Pts',(-0.359809398953095,0.190651033176329,
-0.421330460721335));
#33447=CARTESIAN_POINT('Ctrl Pts',(-0.297175326236494,0.261759452748588,
-0.42420368331354));
#33448=CARTESIAN_POINT('Ctrl Pts',(-0.211552007063425,0.358967547972998,
-0.428131495196073));
#33449=CARTESIAN_POINT('Ctrl Pts',(-0.0736307456486751,0.41011030892357,
-0.432059307078606));
#33450=CARTESIAN_POINT('Ctrl Pts',(0.0546695748141089,0.392227514609258,
-0.435987118961139));
#33451=CARTESIAN_POINT('Ctrl Pts',(0.182969895276892,0.374344720294945,
-0.439914930843672));
#33452=CARTESIAN_POINT('Ctrl Pts',(0.301649274787709,0.287436370715749,
-0.443842742726204));
#33453=CARTESIAN_POINT('Ctrl Pts',(0.357427352060231,0.170519423016928,
-0.447770554608737));
#33454=CARTESIAN_POINT('Ctrl Pts',(0.413205429332753,0.0536024753181058,
-0.45169836649127));
#33455=CARTESIAN_POINT('Ctrl Pts',(0.40608220436698,-0.0933230705003415,
-0.455626178373802));
#33456=CARTESIAN_POINT('Ctrl Pts',(0.339255604225498,-0.204295914371732,
-0.459553990256335));
#33457=CARTESIAN_POINT('Ctrl Pts',(0.272429004084016,-0.315268758243122,
-0.463481802138868));
#33458=CARTESIAN_POINT('Ctrl Pts',(0.145899028766824,-0.390288900167456,
-0.467409614021401));
#33459=CARTESIAN_POINT('Ctrl Pts',(0.0164705151944307,-0.395676519085635,
-0.471337425903934));
#33460=CARTESIAN_POINT('Ctrl Pts',(-0.112957998377962,-0.401064138003814,
-0.475265237786467));
#33461=CARTESIAN_POINT('Ctrl Pts',(-0.245285050205555,-0.33681923391584,
-0.479193049668999));
#33462=CARTESIAN_POINT('Ctrl Pts',(-0.321103242324281,-0.231784152597038,
-0.483120861551532));
#33463=CARTESIAN_POINT('Ctrl Pts',(-0.369123434363212,-0.165259158597507,
-0.485608579546663));
#33464=CARTESIAN_POINT('Ctrl Pts',(-0.394475403221431,-0.0823714058055866,
-0.488096297541793));
#33465=CARTESIAN_POINT('Ctrl Pts',(-0.394956676078496,0.000245896443633459,
-0.490584015536923));
#33466=CARTESIAN_POINT('Ctrl Pts',(-0.394961414894976,0.000248589851300403,
-0.501115984463076));
#33467=CARTESIAN_POINT('Ctrl Pts',(-0.394473038577377,-0.0826114662579111,
-0.498620880696199));
#33468=CARTESIAN_POINT('Ctrl Pts',(-0.368958940221529,-0.165746803632547,
-0.496125776929321));
#33469=CARTESIAN_POINT('Ctrl Pts',(-0.320672414820748,-0.232379781053294,
-0.493630673162443));
#33470=CARTESIAN_POINT('Ctrl Pts',(-0.244659388527761,-0.337273935739795,
-0.489702861279911));
#33471=CARTESIAN_POINT('Ctrl Pts',(-0.11221332106507,-0.401273092416749,
-0.485775049397377));
#33472=CARTESIAN_POINT('Ctrl Pts',(0.0172049583135898,-0.395645232092361,
-0.481847237514845));
#33473=CARTESIAN_POINT('Ctrl Pts',(0.14662323769225,-0.390017371767973,
-0.477919425632312));
#33474=CARTESIAN_POINT('Ctrl Pts',(0.273013728986881,-0.314762494442241,
-0.473991613749779));
#33475=CARTESIAN_POINT('Ctrl Pts',(0.339634215735493,-0.203665804142061,
-0.470063801867247));
#33476=CARTESIAN_POINT('Ctrl Pts',(0.406254702484105,-0.092569113841881,
-0.466135989984714));
#33477=CARTESIAN_POINT('Ctrl Pts',(0.413105184686698,0.0543693894327481,
-0.462208178102181));
#33478=CARTESIAN_POINT('Ctrl Pts',(0.357110181438081,0.171182588438861,
-0.458280366219648));
#33479=CARTESIAN_POINT('Ctrl Pts',(0.301115178189463,0.287995787444972,
-0.454352554337115));
#33480=CARTESIAN_POINT('Ctrl Pts',(0.182274689489637,0.374683682182567,
-0.450424742454583));
#33481=CARTESIAN_POINT('Ctrl Pts',(0.0539414055779334,0.392328287325614,
-0.44649693057205));
#33482=CARTESIAN_POINT('Ctrl Pts',(-0.0743918783337699,0.409972892468661,
-0.442569118689517));
#33483=CARTESIAN_POINT('Ctrl Pts',(-0.212217957457349,0.35857420801716,
-0.438641306806984));
#33484=CARTESIAN_POINT('Ctrl Pts',(-0.297660680088029,0.261207350206704,
-0.434713494924451));
#33485=CARTESIAN_POINT('Ctrl Pts',(-0.360001980506246,0.190165881177487,
-0.431847658103993));
#33486=CARTESIAN_POINT('Ctrl Pts',(-0.394456725068691,0.0946530128377653,
-0.428981821283535));
#33487=CARTESIAN_POINT('Ctrl Pts',(-0.395260053944926,-0.00033663270935099,
-0.426115984463076));
#33488=CARTESIAN_POINT('Origin',(0.,0.,-0.48));
#33489=CARTESIAN_POINT('',(-0.395875933213339,0.00020569453982186,-0.340584015536923));
#33490=CARTESIAN_POINT('',(-0.395880924684652,0.000202294883939828,-0.351115984463076));
#33491=CARTESIAN_POINT('',(-0.3954,-4.84225344382863E-17,-0.48));
#33492=CARTESIAN_POINT('Ctrl Pts',(-0.395875933213339,0.00020569453982186,
-0.340584015536923));
#33493=CARTESIAN_POINT('Ctrl Pts',(-0.39595581585693,0.0127020976124944,
-0.340962554951399));
#33494=CARTESIAN_POINT('Ctrl Pts',(-0.395414255679657,0.0251914927215432,
-0.341341094365876));
#33495=CARTESIAN_POINT('Ctrl Pts',(-0.394228317772475,0.0376193978231643,
-0.341719633780352));
#33496=CARTESIAN_POINT('Ctrl Pts',(-0.38192275373967,0.166574194777889,
-0.345647445662884));
#33497=CARTESIAN_POINT('Ctrl Pts',(-0.30023952618032,0.288908599922735,
-0.349575257545417));
#33498=CARTESIAN_POINT('Ctrl Pts',(-0.185849806556546,0.349701351197546,
-0.35350306942795));
#33499=CARTESIAN_POINT('Ctrl Pts',(-0.0714600869327725,0.410494102472356,
-0.357430881310483));
#33500=CARTESIAN_POINT('Ctrl Pts',(0.0756361247554245,0.409745199877132,
-0.361358693193016));
#33501=CARTESIAN_POINT('Ctrl Pts',(0.189400909071263,0.347790858520418,
-0.365286505075549));
#33502=CARTESIAN_POINT('Ctrl Pts',(0.303165693387101,0.285836517163703,
-0.369214316958082));
#33503=CARTESIAN_POINT('Ctrl Pts',(0.383599050330581,0.162676737045497,
-0.373142128840614));
#33504=CARTESIAN_POINT('Ctrl Pts',(0.394590929992081,0.0336033271388246,
-0.377069940723147));
#33505=CARTESIAN_POINT('Ctrl Pts',(0.405582809653581,-0.0954700827678465,
-0.38099775260568));
#33506=CARTESIAN_POINT('Ctrl Pts',(0.347133212033103,-0.230457122462983,
-0.384925564488213));
#33507=CARTESIAN_POINT('Ctrl Pts',(0.245482716505811,-0.310756209147683,
-0.388853376370745));
#33508=CARTESIAN_POINT('Ctrl Pts',(0.143832220978519,-0.391055295832382,
-0.392781188253278));
#33509=CARTESIAN_POINT('Ctrl Pts',(-0.00101917245558511,-0.416666429506645,
-0.396709000135811));
#33510=CARTESIAN_POINT('Ctrl Pts',(-0.124041341403078,-0.376091652725678,
-0.400636812018344));
#33511=CARTESIAN_POINT('Ctrl Pts',(-0.247063510350573,-0.33551687594471,
-0.404564623900876));
#33512=CARTESIAN_POINT('Ctrl Pts',(-0.348256454811456,-0.228756188708513,
-0.408492435783409));
#33513=CARTESIAN_POINT('Ctrl Pts',(-0.382190238576203,-0.10373913034129,
-0.412420247665942));
#33514=CARTESIAN_POINT('Ctrl Pts',(-0.391301215885916,-0.0701729477426301,
-0.413474836956269));
#33515=CARTESIAN_POINT('Ctrl Pts',(-0.395563588278611,-0.0352906926578339,
-0.414529426246596));
#33516=CARTESIAN_POINT('Ctrl Pts',(-0.395266933374857,-0.000337325613274597,
-0.415584015536924));
#33517=CARTESIAN_POINT('Ctrl Pts',(-0.395260053944926,-0.00033663270935099,
-0.426115984463076));
#33518=CARTESIAN_POINT('Ctrl Pts',(-0.39555773845617,-0.0355363461076123,
-0.425054009401002));
#33519=CARTESIAN_POINT('Ctrl Pts',(-0.39123449647611,-0.0706642118877601,
-0.423992034338928));
#33520=CARTESIAN_POINT('Ctrl Pts',(-0.381996983921461,-0.104448382212464,
-0.422930059276853));
#33521=CARTESIAN_POINT('Ctrl Pts',(-0.347831198986433,-0.229402225651767,
-0.41900224739432));
#33522=CARTESIAN_POINT('Ctrl Pts',(-0.246440262978595,-0.335974881360961,
-0.415074435511788));
#33523=CARTESIAN_POINT('Ctrl Pts',(-0.123342999167154,-0.376321225588517,
-0.411146623629255));
#33524=CARTESIAN_POINT('Ctrl Pts',(-0.000245735355712692,-0.416667569816073,
-0.407218811746722));
#33525=CARTESIAN_POINT('Ctrl Pts',(0.144557856259332,-0.390787602561992,
-0.403290999864189));
#33526=CARTESIAN_POINT('Ctrl Pts',(0.246059113610558,-0.310299972415847,
-0.399363187981656));
#33527=CARTESIAN_POINT('Ctrl Pts',(0.347560370961784,-0.229812342269703,
-0.395435376099124));
#33528=CARTESIAN_POINT('Ctrl Pts',(0.405759294049192,-0.0947170492314976,
-0.391507564216591));
#33529=CARTESIAN_POINT('Ctrl Pts',(0.394527842253011,0.0343357242411698,
-0.387579752334058));
#33530=CARTESIAN_POINT('Ctrl Pts',(0.383296390456831,0.163388497713835,
-0.383651940451526));
#33531=CARTESIAN_POINT('Ctrl Pts',(0.302634563777064,0.286398751620962,
-0.379724128568993));
#33532=CARTESIAN_POINT('Ctrl Pts',(0.188754982175704,0.34814180584345,-0.37579631668646));
#33533=CARTESIAN_POINT('Ctrl Pts',(0.0748754005743428,0.409884860065939,
-0.371868504803927));
#33534=CARTESIAN_POINT('Ctrl Pts',(-0.0722219359486128,0.410360714603788,
-0.367940692921395));
#33535=CARTESIAN_POINT('Ctrl Pts',(-0.186498602970298,0.349355737554315,
-0.364012881038862));
#33536=CARTESIAN_POINT('Ctrl Pts',(-0.300775269991983,0.288350760504841,
-0.360085069156329));
#33537=CARTESIAN_POINT('Ctrl Pts',(-0.382231267512398,0.165864951868046,
-0.356157257273796));
#33538=CARTESIAN_POINT('Ctrl Pts',(-0.394297437564028,0.0368875453552563,
-0.352229445391263));
#33539=CARTESIAN_POINT('Ctrl Pts',(-0.395437615124049,0.0246999875778991,
-0.351858291748534));
#33540=CARTESIAN_POINT('Ctrl Pts',(-0.395958206245996,0.0124544658863471,
-0.351487138105805));
#33541=CARTESIAN_POINT('Ctrl Pts',(-0.395880924684652,0.000202294883939828,
-0.351115984463076));
#33542=CARTESIAN_POINT('Origin',(0.,0.,-0.48));
#33543=CARTESIAN_POINT('',(-0.394796739701267,7.87737235064534E-5,-0.265584015536923));
#33544=CARTESIAN_POINT('',(-0.394798228541794,8.25237670084469E-5,-0.276115984463076));
#33545=CARTESIAN_POINT('',(-0.3954,-4.84225344382863E-17,-0.48));
#33546=CARTESIAN_POINT('Ctrl Pts',(-0.394796739701267,7.87737235064534E-5,
-0.265584015536923));
#33547=CARTESIAN_POINT('Ctrl Pts',(-0.394906225968879,0.0603056496953535,
-0.267395683656203));
#33548=CARTESIAN_POINT('Ctrl Pts',(-0.381947457713303,0.12048784623346,
-0.269207351775482));
#33549=CARTESIAN_POINT('Ctrl Pts',(-0.355672556193802,0.17414998820835,
-0.271019019894762));
#33550=CARTESIAN_POINT('Ctrl Pts',(-0.298706896036511,0.290492930189886,
-0.274946831777295));
#33551=CARTESIAN_POINT('Ctrl Pts',(-0.179148748818222,0.376188354397569,
-0.278874643659828));
#33552=CARTESIAN_POINT('Ctrl Pts',(-0.0506729928961993,0.392763839202375,
-0.28280245554236));
#33553=CARTESIAN_POINT('Ctrl Pts',(0.0778027630258239,0.409339324007181,
-0.286730267424893));
#33554=CARTESIAN_POINT('Ctrl Pts',(0.215196127651582,0.356794869409109,
-0.290658079307426));
#33555=CARTESIAN_POINT('Ctrl Pts',(0.299825213644828,0.258719977794535,
-0.294585891189959));
#33556=CARTESIAN_POINT('Ctrl Pts',(0.384454299638073,0.160645086179963,
-0.298513703072491));
#33557=CARTESIAN_POINT('Ctrl Pts',(0.416319106998808,0.0170397575488902,
-0.302441514955024));
#33558=CARTESIAN_POINT('Ctrl Pts',(0.381114130844172,-0.107625298583498,
-0.306369326837557));
#33559=CARTESIAN_POINT('Ctrl Pts',(0.345909154689534,-0.23229035471589,
-0.31029713872009));
#33560=CARTESIAN_POINT('Ctrl Pts',(0.243634395019522,-0.338015138349596,
-0.314224950602622));
#33561=CARTESIAN_POINT('Ctrl Pts',(0.12020546215663,-0.377335172612692,
-0.318152762485155));
#33562=CARTESIAN_POINT('Ctrl Pts',(-0.00322347070625931,-0.416655206875788,
-0.322080574367688));
#33563=CARTESIAN_POINT('Ctrl Pts',(-0.147806576762028,-0.389570491768276,
-0.326008386250221));
#33564=CARTESIAN_POINT('Ctrl Pts',(-0.248634179536782,-0.30824053983222,
-0.329936198132754));
#33565=CARTESIAN_POINT('Ctrl Pts',(-0.339744610802606,-0.234748690459619,
-0.33348547060081));
#33566=CARTESIAN_POINT('Ctrl Pts',(-0.39512693520486,-0.116963450017949,
-0.337034743068867));
#33567=CARTESIAN_POINT('Ctrl Pts',(-0.395875933213339,0.00020569453982186,
-0.340584015536923));
#33568=CARTESIAN_POINT('Ctrl Pts',(-0.395880924684652,0.000202294883939828,
-0.351115984463076));
#33569=CARTESIAN_POINT('Ctrl Pts',(-0.395140357786489,-0.11720672373916,
-0.347559326223272));
#33570=CARTESIAN_POINT('Ctrl Pts',(-0.33949812433168,-0.235226337657232,
-0.344002667983469));
#33571=CARTESIAN_POINT('Ctrl Pts',(-0.248061560911564,-0.30870150999079,
-0.340446009743665));
#33572=CARTESIAN_POINT('Ctrl Pts',(-0.147083171624631,-0.389844154435259,
-0.336518197861132));
#33573=CARTESIAN_POINT('Ctrl Pts',(-0.00245005046792381,-0.416660438935413,
-0.332590385978599));
#33574=CARTESIAN_POINT('Ctrl Pts',(0.120905672129734,-0.37711136116329,
-0.328662574096066));
#33575=CARTESIAN_POINT('Ctrl Pts',(0.244261394727393,-0.337562283391168,
-0.324734762213533));
#33576=CARTESIAN_POINT('Ctrl Pts',(0.346339718766002,-0.231647843346768,
-0.320806950331001));
#33577=CARTESIAN_POINT('Ctrl Pts',(0.381313222445306,-0.106917662992341,
-0.316879138448468));
#33578=CARTESIAN_POINT('Ctrl Pts',(0.41628672612461,0.0178125173620851,
-0.312951326565936));
#33579=CARTESIAN_POINT('Ctrl Pts',(0.384155409444609,0.161358438026538,
-0.309023514683403));
#33580=CARTESIAN_POINT('Ctrl Pts',(0.299344425008715,0.259276060389882,
-0.30509570280087));
#33581=CARTESIAN_POINT('Ctrl Pts',(0.214533440572821,0.357193682753226,
-0.301167890918337));
#33582=CARTESIAN_POINT('Ctrl Pts',(0.0770427883810332,0.409483006815461,
-0.297240079035804));
#33583=CARTESIAN_POINT('Ctrl Pts',(-0.0514019676604196,0.392669069304711,
-0.293312267153272));
#33584=CARTESIAN_POINT('Ctrl Pts',(-0.179846723701874,0.375855131793961,
-0.289384455270739));
#33585=CARTESIAN_POINT('Ctrl Pts',(-0.299245583592994,0.289937932710224,
-0.285456643388206));
#33586=CARTESIAN_POINT('Ctrl Pts',(-0.355995179884672,0.173489458377813,
-0.281528831505673));
#33587=CARTESIAN_POINT('Ctrl Pts',(-0.382063713175179,0.119997607719336,
-0.279724549158141));
#33588=CARTESIAN_POINT('Ctrl Pts',(-0.394912485224089,0.0600632843804217,
-0.277920266810608));
#33589=CARTESIAN_POINT('Ctrl Pts',(-0.394798228541794,8.25237670084469E-5,
-0.276115984463076));
#33590=CARTESIAN_POINT('Origin',(0.,0.,-0.48));
#33591=CARTESIAN_POINT('',(-0.395622884157063,-0.00031191406896286,-0.190584015536923));
#33592=CARTESIAN_POINT('',(-0.395615927747866,-0.00031357059932876,-0.201115984463076));
#33593=CARTESIAN_POINT('',(-0.3954,-4.84225344382863E-17,-0.48));
#33594=CARTESIAN_POINT('Ctrl Pts',(-0.395622884157063,-0.00031191406896286,
-0.190584015536923));
#33595=CARTESIAN_POINT('Ctrl Pts',(-0.394695938484083,0.106985189615806,
-0.193828812361006));
#33596=CARTESIAN_POINT('Ctrl Pts',(-0.349385427645315,0.214972363562661,
-0.197073609185089));
#33597=CARTESIAN_POINT('Ctrl Pts',(-0.271471059019966,0.288330801125965,
-0.200318406009172));
#33598=CARTESIAN_POINT('Ctrl Pts',(-0.177156068128913,0.377130858068399,
-0.204246217891704));
#33599=CARTESIAN_POINT('Ctrl Pts',(-0.0350666671734208,0.41518945175117,
-0.208174029774237));
#33600=CARTESIAN_POINT('Ctrl Pts',(0.0910070087554293,0.385420430263643,
-0.21210184165677));
#33601=CARTESIAN_POINT('Ctrl Pts',(0.217080684684278,0.355651408776116,
-0.216029653539303));
#33602=CARTESIAN_POINT('Ctrl Pts',(0.327138635586484,0.258054772118293,
-0.219957465421836));
#33603=CARTESIAN_POINT('Ctrl Pts',(0.37177103208318,0.136445909161074,-0.223885277304369));
#33604=CARTESIAN_POINT('Ctrl Pts',(0.416403428579877,0.0148370462038541,
-0.227813089186901));
#33605=CARTESIAN_POINT('Ctrl Pts',(0.395610270671062,-0.130784043052762,
-0.231740901069434));
#33606=CARTESIAN_POINT('Ctrl Pts',(0.318726518102726,-0.235041682158158,
-0.235668712951967));
#33607=CARTESIAN_POINT('Ctrl Pts',(0.241842765534391,-0.339299321263555,
-0.2395965248345));
#33608=CARTESIAN_POINT('Ctrl Pts',(0.108868418306535,-0.402193510217731,
-0.243524336717033));
#33609=CARTESIAN_POINT('Ctrl Pts',(-0.0204985275777863,-0.39548830038016,
-0.247452148599566));
#33610=CARTESIAN_POINT('Ctrl Pts',(-0.149865473462107,-0.388783090542588,
-0.251379960482098));
#33611=CARTESIAN_POINT('Ctrl Pts',(-0.275625018002894,-0.312478481913271,
-0.255307772364631));
#33612=CARTESIAN_POINT('Ctrl Pts',(-0.34131820372514,-0.200830947720919,
-0.259235584247163));
#33613=CARTESIAN_POINT('Ctrl Pts',(-0.37671099477824,-0.140679840633938,
-0.261351728010417));
#33614=CARTESIAN_POINT('Ctrl Pts',(-0.394668852766622,-0.0702700537530919,
-0.26346787177367));
#33615=CARTESIAN_POINT('Ctrl Pts',(-0.394796739701267,7.87737235064534E-5,
-0.265584015536923));
#33616=CARTESIAN_POINT('Ctrl Pts',(-0.394798228541794,8.25237670084469E-5,
-0.276115984463076));
#33617=CARTESIAN_POINT('Ctrl Pts',(-0.394663755442417,-0.0705111484864399,
-0.273992454928076));
#33618=CARTESIAN_POINT('Ctrl Pts',(-0.376573096370534,-0.141169144930958,
-0.271868925393075));
#33619=CARTESIAN_POINT('Ctrl Pts',(-0.340944796447611,-0.201464155788848,
-0.269745395858075));
#33620=CARTESIAN_POINT('Ctrl Pts',(-0.275044484026637,-0.312989546042017,
-0.265817583975542));
#33621=CARTESIAN_POINT('Ctrl Pts',(-0.149143526492451,-0.389060576967273,
-0.261889772093009));
#33622=CARTESIAN_POINT('Ctrl Pts',(-0.019764367298066,-0.395525637632012,
-0.257961960210476));
#33623=CARTESIAN_POINT('Ctrl Pts',(0.109614791896319,-0.401990698296751,
-0.254034148327944));
#33624=CARTESIAN_POINT('Ctrl Pts',(0.242472152750905,-0.338849788700974,
-0.250106336445411));
#33625=CARTESIAN_POINT('Ctrl Pts',(0.31916223861105,-0.234449622972972,
-0.246178524562878));
#33626=CARTESIAN_POINT('Ctrl Pts',(0.395852324471197,-0.130049457244968,
-0.242250712680345));
#33627=CARTESIAN_POINT('Ctrl Pts',(0.416375135336902,0.0156099646152614,
-0.238322900797812));
#33628=CARTESIAN_POINT('Ctrl Pts',(0.37151708387966,0.137135760428241,-0.23439508891528));
#33629=CARTESIAN_POINT('Ctrl Pts',(0.326659032422418,0.258661556241219,
-0.230467277032747));
#33630=CARTESIAN_POINT('Ctrl Pts',(0.216420118642233,0.356053726006946,
-0.226539465150214));
#33631=CARTESIAN_POINT('Ctrl Pts',(0.0902914106015626,0.385588668383179,
-0.222611653267682));
#33632=CARTESIAN_POINT('Ctrl Pts',(-0.0358372974391088,0.415123610759413,
-0.218683841385149));
#33633=CARTESIAN_POINT('Ctrl Pts',(-0.177855799740265,0.376801325746151,
-0.214756029502616));
#33634=CARTESIAN_POINT('Ctrl Pts',(-0.272005784099203,0.287826360424576,
-0.210828217620083));
#33635=CARTESIAN_POINT('Ctrl Pts',(-0.349606801932139,0.214490736232845,
-0.207590806567747));
#33636=CARTESIAN_POINT('Ctrl Pts',(-0.394688285862518,0.106744154164166,
-0.204353395515412));
#33637=CARTESIAN_POINT('Ctrl Pts',(-0.395615927747866,-0.00031357059932876,
-0.201115984463076));
#33638=CARTESIAN_POINT('Origin',(0.,0.,-0.48));
#33639=CARTESIAN_POINT('',(-0.395559352324906,0.000325232430651398,-0.115584015536923));
#33640=CARTESIAN_POINT('',(-0.395566345080525,0.000324025114679023,-0.126115984463076));
#33641=CARTESIAN_POINT('',(-0.3954,-4.84225344382863E-17,-0.48));
#33642=CARTESIAN_POINT('Ctrl Pts',(-0.395559352324906,0.000325232430651398,
-0.115584015536923));
#33643=CARTESIAN_POINT('Ctrl Pts',(-0.395778471079392,0.0251397697442085,
-0.116334129183277));
#33644=CARTESIAN_POINT('Ctrl Pts',(-0.393638970125572,0.0499166998589586,
-0.11708424282963));
#33645=CARTESIAN_POINT('Ctrl Pts',(-0.389002685395281,0.0742173137443584,
-0.117834356475983));
#33646=CARTESIAN_POINT('Ctrl Pts',(-0.364725758368326,0.20146235246073,
-0.121762168358516));
#33647=CARTESIAN_POINT('Ctrl Pts',(-0.27199020820128,0.315647408351251,
-0.125689980241049));
#33648=CARTESIAN_POINT('Ctrl Pts',(-0.152429834240862,0.365508475309613,
-0.129617792123582));
#33649=CARTESIAN_POINT('Ctrl Pts',(-0.0328694602804443,0.415369542267976,
-0.133545604006115));
#33650=CARTESIAN_POINT('Ctrl Pts',(0.113515737473344,0.400906620294181,
-0.137473415888647));
#33651=CARTESIAN_POINT('Ctrl Pts',(0.221007441079253,0.328613450240116,
-0.14140122777118));
#33652=CARTESIAN_POINT('Ctrl Pts',(0.328499144685164,0.256320280186051,
-0.145329039653713));
#33653=CARTESIAN_POINT('Ctrl Pts',(0.397097354143193,0.126196862051714,
-0.149256851536246));
#33654=CARTESIAN_POINT('Ctrl Pts',(0.396005127209871,-0.00333908159127506,
-0.153184663418779));
#33655=CARTESIAN_POINT('Ctrl Pts',(0.394912900276549,-0.132875025234262,
-0.157112475301311));
#33656=CARTESIAN_POINT('Ctrl Pts',(0.324130236951877,-0.261823494385903,
-0.161040287183844));
#33657=CARTESIAN_POINT('Ctrl Pts',(0.215434677460811,-0.332293691977232,
-0.164968099066377));
#33658=CARTESIAN_POINT('Ctrl Pts',(0.106739117969747,-0.40276388956856,
-0.16889591094891));
#33659=CARTESIAN_POINT('Ctrl Pts',(-0.0398693376877085,-0.414755815599578,
-0.172823722831442));
#33660=CARTESIAN_POINT('Ctrl Pts',(-0.158571801886283,-0.362885871046767,
-0.176751534713975));
#33661=CARTESIAN_POINT('Ctrl Pts',(-0.27727426608486,-0.311015926493954,
-0.180679346596508));
#33662=CARTESIAN_POINT('Ctrl Pts',(-0.368070738824554,-0.195284111357307,
-0.184607158479041));
#33663=CARTESIAN_POINT('Ctrl Pts',(-0.390198684781093,-0.0676474436879351,
-0.188534970361573));
#33664=CARTESIAN_POINT('Ctrl Pts',(-0.394046557528791,-0.0454524484499415,
-0.189217985420023));
#33665=CARTESIAN_POINT('Ctrl Pts',(-0.395818002029563,-0.0228974691955075,
-0.189901000478473));
#33666=CARTESIAN_POINT('Ctrl Pts',(-0.395622884157063,-0.00031191406896286,
-0.190584015536923));
#33667=CARTESIAN_POINT('Ctrl Pts',(-0.395615927747866,-0.00031357059932876,
-0.201115984463076));
#33668=CARTESIAN_POINT('Ctrl Pts',(-0.395813753948313,-0.0231443884537417,
-0.200425583632879));
#33669=CARTESIAN_POINT('Ctrl Pts',(-0.394003526001132,-0.0459438780543778,
-0.199735182802682));
#33670=CARTESIAN_POINT('Ctrl Pts',(-0.390072407059393,-0.0683716192899147,
-0.199044781972485));
#33671=CARTESIAN_POINT('Ctrl Pts',(-0.367707579243926,-0.195966988052947,
-0.195116970089952));
#33672=CARTESIAN_POINT('Ctrl Pts',(-0.276696457196274,-0.311530079949128,
-0.191189158207419));
#33673=CARTESIAN_POINT('Ctrl Pts',(-0.157897917538397,-0.363179578141115,
-0.187261346324886));
#33674=CARTESIAN_POINT('Ctrl Pts',(-0.0390993778805183,-0.414829076333103,
-0.183333534442354));
#33675=CARTESIAN_POINT('Ctrl Pts',(0.107486579387586,-0.402564980820896,
-0.179405722559821));
#33676=CARTESIAN_POINT('Ctrl Pts',(0.216051120986117,-0.331893167348008,
-0.175477910677288));
#33677=CARTESIAN_POINT('Ctrl Pts',(0.324615662584646,-0.261221353875121,
-0.171550098794755));
#33678=CARTESIAN_POINT('Ctrl Pts',(0.395158788513602,-0.132141822441553,
-0.167622286912222));
#33679=CARTESIAN_POINT('Ctrl Pts',(0.396010585569408,-0.00260404166427942,
-0.16369447502969));
#33680=CARTESIAN_POINT('Ctrl Pts',(0.396862382625215,0.126933739112996,
-0.159766663147157));
#33681=CARTESIAN_POINT('Ctrl Pts',(0.328022850807872,0.256929769233978,
-0.155838851264624));
#33682=CARTESIAN_POINT('Ctrl Pts',(0.220397103955469,0.329023195087183,
-0.151911039382091));
#33683=CARTESIAN_POINT('Ctrl Pts',(0.112771357103067,0.401116620940388,
-0.147983227499559));
#33684=CARTESIAN_POINT('Ctrl Pts',(-0.0336406047843918,0.415307442525814,
-0.144055415617026));
#33685=CARTESIAN_POINT('Ctrl Pts',(-0.15310812608344,0.365224690280065,
-0.140127603734493));
#33686=CARTESIAN_POINT('Ctrl Pts',(-0.272575647382488,0.315141938034316,
-0.13619979185196));
#33687=CARTESIAN_POINT('Ctrl Pts',(-0.365098728093125,0.200785611957391,
-0.132271979969427));
#33688=CARTESIAN_POINT('Ctrl Pts',(-0.389139571160733,0.0734954365042287,
-0.128344168086895));
#33689=CARTESIAN_POINT('Ctrl Pts',(-0.393685563893927,0.0494255563012018,
-0.127601440212289));
#33690=CARTESIAN_POINT('Ctrl Pts',(-0.395782854098394,0.0248932036270088,
-0.126858712337682));
#33691=CARTESIAN_POINT('Ctrl Pts',(-0.395566345080525,0.000324025114679023,
-0.126115984463076));
#33692=CARTESIAN_POINT('Origin',(0.,0.,-0.48));
#33693=CARTESIAN_POINT('',(-0.394794988713166,-8.02750947288822E-5,-0.0405840155369234));
#33694=CARTESIAN_POINT('',(-0.39480767064478,-0.000104727820695843,-0.0511159844630761));
#33695=CARTESIAN_POINT('',(-0.3954,-4.84225344382863E-17,-0.48));
#33696=CARTESIAN_POINT('Ctrl Pts',(-0.394794988713166,-8.02750947288822E-5,
-0.0405840155369234));
#33697=CARTESIAN_POINT('Ctrl Pts',(-0.394615005116812,0.0724759759833135,
-0.0427672578880801));
#33698=CARTESIAN_POINT('Ctrl Pts',(-0.37544474313299,0.145114666223604,
-0.0449505002392368));
#33699=CARTESIAN_POINT('Ctrl Pts',(-0.337893742543562,0.206539063180415,
-0.0471337425903935));
#33700=CARTESIAN_POINT('Ctrl Pts',(-0.270336759582872,0.317046023672708,
-0.0510615544729262));
#33701=CARTESIAN_POINT('Ctrl Pts',(-0.14328752260418,0.391256097572554,
-0.054989366355459));
#33702=CARTESIAN_POINT('Ctrl Pts',(-0.01382092735515,0.395787669078235,
-0.0589171782379918));
#33703=CARTESIAN_POINT('Ctrl Pts',(0.11564566789388,0.400319240583916,-0.0628449901205246));
#33704=CARTESIAN_POINT('Ctrl Pts',(0.24752962141325,0.335172309695432,-0.0667728020030573));
#33705=CARTESIAN_POINT('Ctrl Pts',(0.322641754051717,0.229628399641421,
-0.07070061388559));
#33706=CARTESIAN_POINT('Ctrl Pts',(0.397753886690185,0.124084489587409,
-0.0746284257681228));
#33707=CARTESIAN_POINT('Ctrl Pts',(0.41609419844775,-0.0218563996321296,
-0.0785562376506555));
#33708=CARTESIAN_POINT('Ctrl Pts',(0.369418829098776,-0.142692926762401,
-0.0824840495331883));
#33709=CARTESIAN_POINT('Ctrl Pts',(0.322743459749801,-0.263529453892673,
-0.0864118614157211));
#33710=CARTESIAN_POINT('Ctrl Pts',(0.211052409294286,-0.359261618933676,
-0.090339673298254));
#33711=CARTESIAN_POINT('Ctrl Pts',(0.0844939542274045,-0.38690169880114,
-0.0942674851807868));
#33712=CARTESIAN_POINT('Ctrl Pts',(-0.042064500839475,-0.414541778668603,
-0.0981952970633196));
#33713=CARTESIAN_POINT('Ctrl Pts',(-0.183490360517721,-0.37408977336253,
-0.102123108945852));
#33714=CARTESIAN_POINT('Ctrl Pts',(-0.276294138413411,-0.283711259938383,
-0.106050920828385));
#33715=CARTESIAN_POINT('Ctrl Pts',(-0.351374720210459,-0.210592777871152,
-0.109228619064565));
#33716=CARTESIAN_POINT('Ctrl Pts',(-0.394631101941742,-0.104796320598328,
-0.112406317300744));
#33717=CARTESIAN_POINT('Ctrl Pts',(-0.395559352324906,0.000325232430651398,
-0.115584015536923));
#33718=CARTESIAN_POINT('Ctrl Pts',(-0.395566345080525,0.000324025114679023,
-0.126115984463076));
#33719=CARTESIAN_POINT('Ctrl Pts',(-0.394637876614533,-0.105037440696735,
-0.122930900455149));
#33720=CARTESIAN_POINT('Ctrl Pts',(-0.351158580959819,-0.211076134618309,
-0.119745816447223));
#33721=CARTESIAN_POINT('Ctrl Pts',(-0.275767342730863,-0.284224269941031,
-0.116560732439296));
#33722=CARTESIAN_POINT('Ctrl Pts',(-0.182795665808806,-0.374429776103722,
-0.112632920556764));
#33723=CARTESIAN_POINT('Ctrl Pts',(-0.0412937065401148,-0.414616763599703,
-0.108705108674231));
#33724=CARTESIAN_POINT('Ctrl Pts',(0.085212636995385,-0.386742913751592,
-0.104777296791698));
#33725=CARTESIAN_POINT('Ctrl Pts',(0.211718980530884,-0.358869063903481,
-0.100849484909165));
#33726=CARTESIAN_POINT('Ctrl Pts',(0.32322970833319,-0.262934376711279,
-0.0969216730266324));
#33727=CARTESIAN_POINT('Ctrl Pts',(0.369681792863869,-0.14200931744245,
-0.0929938611440997));
#33728=CARTESIAN_POINT('Ctrl Pts',(0.416133877394547,-0.0210842581736197,
-0.0890660492615669));
#33729=CARTESIAN_POINT('Ctrl Pts',(0.397527318653598,0.124831173171839,
-0.0851382373790342));
#33730=CARTESIAN_POINT('Ctrl Pts',(0.322217300233705,0.230231435304264,
-0.0812104254965014));
#33731=CARTESIAN_POINT('Ctrl Pts',(0.246907281813811,0.335631697436688,
-0.0772826136139687));
#33732=CARTESIAN_POINT('Ctrl Pts',(0.114893803714973,0.40051679035608,-0.0733548017314358));
#33733=CARTESIAN_POINT('Ctrl Pts',(-0.0145601156695766,0.395752615374949,
-0.0694269898489031));
#33734=CARTESIAN_POINT('Ctrl Pts',(-0.144014035054129,0.390988440393817,
-0.0654991779663702));
#33735=CARTESIAN_POINT('Ctrl Pts',(-0.270908395724393,0.316574997512162,
-0.0615713660838375));
#33736=CARTESIAN_POINT('Ctrl Pts',(-0.338267890539552,0.205928032203031,
-0.0576435542013047));
#33737=CARTESIAN_POINT('Ctrl Pts',(-0.375582457622321,0.144633872844177,
-0.0554676976218951));
#33738=CARTESIAN_POINT('Ctrl Pts',(-0.394627361076789,0.0722206111356247,
-0.0532918410424856));
#33739=CARTESIAN_POINT('Ctrl Pts',(-0.39480767064478,-0.000104727820695843,
-0.0511159844630761));
#33740=CARTESIAN_POINT('Origin',(0.,0.,-0.953243520205039));
#33741=CARTESIAN_POINT('',(-0.351835822326257,-7.15400518810813E-5,-0.015743520205039));
#33742=CARTESIAN_POINT('',(-0.352300869236444,-9.88871641177669E-6,-0.00095647979495892));
#33743=CARTESIAN_POINT('',(-0.352375,-1.84016574122319E-14,-0.953243520205039));
#33744=CARTESIAN_POINT('',(-0.0878173632231217,-0.341256870028339,-1.11022302462516E-16));
#33745=CARTESIAN_POINT('Ctrl Pts',(-0.351835822326257,-7.15400518810534E-5,
-0.015743520205039));
#33746=CARTESIAN_POINT('Ctrl Pts',(-0.351963992710222,-0.0517404851579902,
-0.0139989506736631));
#33747=CARTESIAN_POINT('Ctrl Pts',(-0.319843451957026,-0.207024739602225,
-0.00875111060531678));
#33748=CARTESIAN_POINT('Ctrl Pts',(-0.187433410478183,-0.315404643562256,
-0.00350327053697048));
#33749=CARTESIAN_POINT('Ctrl Pts',(-0.0877607245812972,-0.341761560210009,
-9.26992857475106E-17));
#33750=CARTESIAN_POINT('',(-0.351244341336214,-0.0282055544935595,-2.22044604925031E-16));
#33751=CARTESIAN_POINT('Origin',(0.,0.,-1.11022302462516E-16));
#33752=CARTESIAN_POINT('Ctrl Pts',(-0.352300869236444,-9.88871641181485E-6,
-0.000956479794958919));
#33753=CARTESIAN_POINT('Ctrl Pts',(-0.352345797709144,-0.00941591104682515,
-0.000637653196639279));
#33754=CARTESIAN_POINT('Ctrl Pts',(-0.351997710417371,-0.0188238340684492,
-0.00031882659831964));
#33755=CARTESIAN_POINT('Ctrl Pts',(-0.351244341336214,-0.0282055544935645,
0.));
#33756=CARTESIAN_POINT('Origin',(0.,0.,-0.953243520205039));
#33757=CARTESIAN_POINT('',(-0.352517012583431,0.000289842634663734,-0.0907435202050393));
#33758=CARTESIAN_POINT('',(-0.351847124287948,-9.33319823582524E-5,-0.0759564797949592));
#33759=CARTESIAN_POINT('',(-0.352375,-1.84016574122319E-14,-0.953243520205039));
#33760=CARTESIAN_POINT('Ctrl Pts',(-0.352517012583431,0.000289842634663726,
-0.0907435202050393));
#33761=CARTESIAN_POINT('Ctrl Pts',(-0.35168976870693,-0.0933930285049049,
-0.08756582196886));
#33762=CARTESIAN_POINT('Ctrl Pts',(-0.265490968213442,-0.304218052429229,
-0.0804603118501481));
#33763=CARTESIAN_POINT('Ctrl Pts',(0.0885494659099983,-0.405484154345161,
-0.0694269898489031));
#33764=CARTESIAN_POINT('Ctrl Pts',(0.387162014500754,-0.149538618257732,
-0.0576435542013047));
#33765=CARTESIAN_POINT('Ctrl Pts',(0.338128119541936,0.240642875207636,
-0.0458601185537062));
#33766=CARTESIAN_POINT('Ctrl Pts',(-0.01447133509682,0.414817000942304,
-0.0340766829061081));
#33767=CARTESIAN_POINT('Ctrl Pts',(-0.303855303328585,0.245786425248945,
-0.0240378167898856));
#33768=CARTESIAN_POINT('Ctrl Pts',(-0.351675423439652,0.0645895853240114,
-0.0179267625561959));
#33769=CARTESIAN_POINT('Ctrl Pts',(-0.351835822326257,-7.15400518810534E-5,
-0.015743520205039));
#33770=CARTESIAN_POINT('Ctrl Pts',(-0.351847124287948,-9.33319823582628E-5,
-0.0759564797949592));
#33771=CARTESIAN_POINT('Ctrl Pts',(-0.351976508103106,-0.0519914558104146,
-0.0742045244918361));
#33772=CARTESIAN_POINT('Ctrl Pts',(-0.317060654848262,-0.2200783548687,
-0.0685247573061803));
#33773=CARTESIAN_POINT('Ctrl Pts',(-0.0593024712652474,-0.410811133390711,
-0.0589171782379917));
#33774=CARTESIAN_POINT('Ctrl Pts',(0.31016609475332,-0.275771257119863,
-0.0471337425903933));
#33775=CARTESIAN_POINT('Ctrl Pts',(0.400971528752744,0.106676728393338,
-0.0353503069427951));
#33776=CARTESIAN_POINT('Ctrl Pts',(0.13207620156309,0.39373277295688,-0.0235668712951966));
#33777=CARTESIAN_POINT('Ctrl Pts',(-0.245564839941522,0.328304388362198,
-0.012102262245918));
#33778=CARTESIAN_POINT('Ctrl Pts',(-0.351792297499737,0.106462395441665,
-0.00456546507917205));
#33779=CARTESIAN_POINT('Ctrl Pts',(-0.352300869236444,-9.88871641181485E-6,
-0.000956479794958919));
#33780=CARTESIAN_POINT('Origin',(0.,0.,-0.953243520205039));
#33781=CARTESIAN_POINT('',(-0.352573631271738,-0.000277973495335076,-0.165743520205039));
#33782=CARTESIAN_POINT('',(-0.352523244430323,0.000288766691396741,-0.150956479794959));
#33783=CARTESIAN_POINT('',(-0.352375,-1.84016574122319E-14,-0.953243520205039));
#33784=CARTESIAN_POINT('Ctrl Pts',(-0.352573631271738,-0.000277973495335138,
-0.165743520205039));
#33785=CARTESIAN_POINT('Ctrl Pts',(-0.352747517615496,-0.0204059072022519,
-0.165060505146589));
#33786=CARTESIAN_POINT('Ctrl Pts',(-0.342090283220367,-0.15609951803055,
-0.160449678205607));
#33787=CARTESIAN_POINT('Ctrl Pts',(-0.166186424962074,-0.380311672880833,
-0.151911039382091));
#33788=CARTESIAN_POINT('Ctrl Pts',(0.225779846375536,-0.348250558046386,
-0.140127603734493));
#33789=CARTESIAN_POINT('Ctrl Pts',(0.415021432028277,-0.00349929236118479,
-0.128344168086895));
#33790=CARTESIAN_POINT('Ctrl Pts',(0.231620111407843,0.344393268071943,
-0.116560732439296));
#33791=CARTESIAN_POINT('Ctrl Pts',(-0.159749266881169,0.383060734919559,
-0.104777296791698));
#33792=CARTESIAN_POINT('Ctrl Pts',(-0.340821595749303,0.160106819675714,
-0.096171559380279));
#33793=CARTESIAN_POINT('Ctrl Pts',(-0.35271228818058,0.0224042143743351,
-0.0914936338513928));
#33794=CARTESIAN_POINT('Ctrl Pts',(-0.352517012583431,0.000289842634663726,
-0.0907435202050393));
#33795=CARTESIAN_POINT('Ctrl Pts',(-0.352523244430323,0.000288766691396772,
-0.150956479794959));
#33796=CARTESIAN_POINT('Ctrl Pts',(-0.351695806201427,-0.0936079113948325,
-0.147771395787033));
#33797=CARTESIAN_POINT('Ctrl Pts',(-0.26516385741625,-0.304644789833165,
-0.140658499896574));
#33798=CARTESIAN_POINT('Ctrl Pts',(0.0893042060071663,-0.40531479967714,
-0.129617792123582));
#33799=CARTESIAN_POINT('Ctrl Pts',(0.387434651449787,-0.148827808786758,
-0.117834356475983));
#33800=CARTESIAN_POINT('Ctrl Pts',(0.33768892962625,0.241285621564956,-0.106050920828385));
#33801=CARTESIAN_POINT('Ctrl Pts',(-0.0152568165427812,0.414759708192197,
-0.0942674851807867));
#33802=CARTESIAN_POINT('Ctrl Pts',(-0.304075372848491,0.245390612282059,
-0.0842360048363115));
#33803=CARTESIAN_POINT('Ctrl Pts',(-0.351686434899936,0.0643620077109535,
-0.0781323363743689));
#33804=CARTESIAN_POINT('Ctrl Pts',(-0.351847124287948,-9.33319823582628E-5,
-0.0759564797949592));
#33805=CARTESIAN_POINT('Origin',(0.,0.,-0.953243520205039));
#33806=CARTESIAN_POINT('',(-0.351837382782584,7.0202050624176E-5,-0.240743520205039));
#33807=CARTESIAN_POINT('',(-0.352567431816273,-0.00027944977225125,-0.225956479794959));
#33808=CARTESIAN_POINT('',(-0.352375,-1.84016574122319E-14,-0.953243520205039));
#33809=CARTESIAN_POINT('Ctrl Pts',(-0.351837382782584,7.02020506242011E-5,
-0.240743520205039));
#33810=CARTESIAN_POINT('Ctrl Pts',(-0.351723411718861,-0.0626236980051817,
-0.238627376441786));
#33811=CARTESIAN_POINT('Ctrl Pts',(-0.306014692059434,-0.241840017228692,
-0.232583420796));
#33812=CARTESIAN_POINT('Ctrl Pts',(-0.0214828697613762,-0.414479711673496,
-0.222611653267681));
#33813=CARTESIAN_POINT('Ctrl Pts',(0.334031816159831,-0.24632842310955,
-0.210828217620083));
#33814=CARTESIAN_POINT('Ctrl Pts',(0.389623538603825,0.142998066471633,
-0.199044781972485));
#33815=CARTESIAN_POINT('Ctrl Pts',(0.095377177077531,0.403928376352516,
-0.187261346324887));
#33816=CARTESIAN_POINT('Ctrl Pts',(-0.262487523267468,0.308074448246341,
-0.176160925735738));
#33817=CARTESIAN_POINT('Ctrl Pts',(-0.351747550134876,0.0953437182368893,
-0.168988317029122));
#33818=CARTESIAN_POINT('Ctrl Pts',(-0.352573631271738,-0.000277973495335138,
-0.165743520205039));
#33819=CARTESIAN_POINT('Ctrl Pts',(-0.352567431816273,-0.000279449772251281,
-0.225956479794959));
#33820=CARTESIAN_POINT('Ctrl Pts',(-0.352743731784361,-0.0206259582230498,
-0.225266078964762));
#33821=CARTESIAN_POINT('Ctrl Pts',(-0.341952418100667,-0.156540578529107,
-0.220647866252033));
#33822=CARTESIAN_POINT('Ctrl Pts',(-0.16548019720029,-0.380619515500736,
-0.21210184165677));
#33823=CARTESIAN_POINT('Ctrl Pts',(0.226425923378982,-0.347830739657686,
-0.200318406009172));
#33824=CARTESIAN_POINT('Ctrl Pts',(0.415027091810056,-0.00272907130485191,
-0.188534970361573));
#33825=CARTESIAN_POINT('Ctrl Pts',(0.230980581763497,0.344822909832333,
-0.176751534713975));
#33826=CARTESIAN_POINT('Ctrl Pts',(-0.160460352000493,0.382762900395039,
-0.164968099066377));
#33827=CARTESIAN_POINT('Ctrl Pts',(-0.340962773002534,0.159666203276401,
-0.156369747426705));
#33828=CARTESIAN_POINT('Ctrl Pts',(-0.352716194266368,0.0221844780679374,
-0.151699207669566));
#33829=CARTESIAN_POINT('Ctrl Pts',(-0.352523244430323,0.000288766691396772,
-0.150956479794959));
#33830=CARTESIAN_POINT('Origin',(0.,0.,-0.953243520205039));
#33831=CARTESIAN_POINT('',(-0.352799145083587,0.000183312123080604,-0.315743520205039));
#33832=CARTESIAN_POINT('',(-0.351838709616628,7.35440374098617E-5,-0.300956479794959));
#33833=CARTESIAN_POINT('',(-0.352375,-1.84016574122319E-14,-0.953243520205039));
#33834=CARTESIAN_POINT('Ctrl Pts',(-0.352799145083587,0.000183312123080604,
-0.315743520205039));
#33835=CARTESIAN_POINT('Ctrl Pts',(-0.352131648439078,-0.104236205614763,
-0.312194247736983));
#33836=CARTESIAN_POINT('Ctrl Pts',(-0.248155783239845,-0.325368532847375,
-0.304717163386393));
#33837=CARTESIAN_POINT('Ctrl Pts',(0.125977747866173,-0.395454868510028,
-0.293312267153272));
#33838=CARTESIAN_POINT('Ctrl Pts',(0.399415292924746,-0.112793482827731,
-0.281528831505673));
#33839=CARTESIAN_POINT('Ctrl Pts',(0.314222868844781,0.271143752956601,
-0.269745395858075));
#33840=CARTESIAN_POINT('Ctrl Pts',(-0.0531063182568973,0.411624422068856,
-0.257961960210477));
#33841=CARTESIAN_POINT('Ctrl Pts',(-0.315348018446608,0.223658028597815,
-0.248294668326131));
#33842=CARTESIAN_POINT('Ctrl Pts',(-0.351934955426869,0.0537435592094025,
-0.242555188324319));
#33843=CARTESIAN_POINT('Ctrl Pts',(-0.351837382782584,7.02020506242011E-5,
-0.240743520205039));
#33844=CARTESIAN_POINT('Ctrl Pts',(-0.351838709616628,7.35440374098409E-5,
-0.300956479794959));
#33845=CARTESIAN_POINT('Ctrl Pts',(-0.351718869054174,-0.0628385582901232,
-0.298832950259959));
#33846=CARTESIAN_POINT('Ctrl Pts',(-0.305776206148664,-0.242280141890258,
-0.292781608842426));
#33847=CARTESIAN_POINT('Ctrl Pts',(-0.0207134553279411,-0.414518842516768,
-0.28280245554236));
#33848=CARTESIAN_POINT('Ctrl Pts',(0.334488460689772,-0.245707931903623,
-0.271019019894762));
#33849=CARTESIAN_POINT('Ctrl Pts',(0.389357394519836,0.14372104213278,-0.259235584247163));
#33850=CARTESIAN_POINT('Ctrl Pts',(0.0946272181670758,0.404104697832314,
-0.247452148599565));
#33851=CARTESIAN_POINT('Ctrl Pts',(-0.262820927742507,0.307650859050363,
-0.236359113782163));
#33852=CARTESIAN_POINT('Ctrl Pts',(-0.351740730224602,0.0951289107829825,
-0.229193890847295));
#33853=CARTESIAN_POINT('Ctrl Pts',(-0.352567431816273,-0.000279449772251281,
-0.225956479794959));
#33854=CARTESIAN_POINT('Origin',(0.,0.,-0.953243520205039));
#33855=CARTESIAN_POINT('',(-0.352256412867894,-0.000300619911437438,-0.390743520205039));
#33856=CARTESIAN_POINT('',(-0.352803593413643,0.000180282396865468,-0.375956479794959));
#33857=CARTESIAN_POINT('',(-0.352375,-1.84016574122319E-14,-0.953243520205039));
#33858=CARTESIAN_POINT('Ctrl Pts',(-0.352256412867894,-0.000300619911437438,
-0.390743520205039));
#33859=CARTESIAN_POINT('Ctrl Pts',(-0.352520787606664,-0.0314505761894478,
-0.389688930914712));
#33860=CARTESIAN_POINT('Ctrl Pts',(-0.334574478215314,-0.178318959414863,
-0.384706529741852));
#33861=CARTESIAN_POINT('Ctrl Pts',(-0.129997826644863,-0.394151634612728,
-0.37579631668646));
#33862=CARTESIAN_POINT('Ctrl Pts',(0.257270836187783,-0.325678772484742,
-0.364012881038862));
#33863=CARTESIAN_POINT('Ctrl Pts',(0.41353925015983,0.0352169643329669,
-0.352229445391263));
#33864=CARTESIAN_POINT('Ctrl Pts',(0.198495971305819,0.364491831701348,
-0.340446009743665));
#33865=CARTESIAN_POINT('Ctrl Pts',(-0.194774344275583,0.366494066541952,
-0.328662574096066));
#33866=CARTESIAN_POINT('Ctrl Pts',(-0.347379815174857,0.137941644433663,
-0.320428410916525));
#33867=CARTESIAN_POINT('Ctrl Pts',(-0.352870335388431,0.0113199333490138,
-0.316122059619516));
#33868=CARTESIAN_POINT('Ctrl Pts',(-0.352799145083587,0.000183312123080604,
-0.315743520205039));
#33869=CARTESIAN_POINT('Ctrl Pts',(-0.352803593413643,0.000180282396865497,
-0.375956479794959));
#33870=CARTESIAN_POINT('Ctrl Pts',(-0.352143610457793,-0.10445300778349,
-0.372399821555156));
#33871=CARTESIAN_POINT('Ctrl Pts',(-0.247793743118397,-0.325783646241757,
-0.36491535143282));
#33872=CARTESIAN_POINT('Ctrl Pts',(0.126711582028227,-0.395220309612058,
-0.353503069427949));
#33873=CARTESIAN_POINT('Ctrl Pts',(0.399623944950114,-0.112051866435688,
-0.341719633780353));
#33874=CARTESIAN_POINT('Ctrl Pts',(0.313718992635124,0.271726538679157,
-0.329936198132753));
#33875=CARTESIAN_POINT('Ctrl Pts',(-0.0538702984580581,0.411525101398655,
-0.318152762485156));
#33876=CARTESIAN_POINT('Ctrl Pts',(-0.315562529348155,0.223216238813576,
-0.308492856372557));
#33877=CARTESIAN_POINT('Ctrl Pts',(-0.351940533588365,0.0535275665997614,
-0.302760762142492));
#33878=CARTESIAN_POINT('Ctrl Pts',(-0.351838709616628,7.35440374098409E-5,
-0.300956479794959));
#33879=CARTESIAN_POINT('Origin',(0.,0.,-0.953243520205039));
#33880=CARTESIAN_POINT('',(-0.351979915865352,0.000219139502586136,-0.46574352020504));
#33881=CARTESIAN_POINT('',(-0.352250282015284,-0.000300002405069166,-0.45095647979496));
#33882=CARTESIAN_POINT('',(-0.352375,-1.84016574122319E-14,-0.953243520205039));
#33883=CARTESIAN_POINT('Ctrl Pts',(-0.351979915865352,0.000219139502586143,
-0.46574352020504));
#33884=CARTESIAN_POINT('Ctrl Pts',(-0.351551012165278,-0.0734082552370908,
-0.463255802209909));
#33885=CARTESIAN_POINT('Ctrl Pts',(-0.293285509062973,-0.263906146917594,
-0.456840272332246));
#33886=CARTESIAN_POINT('Ctrl Pts',(0.0172614319911864,-0.414676969416019,
-0.44649693057205));
#33887=CARTESIAN_POINT('Ctrl Pts',(0.355546713117099,-0.214106237165738,
-0.434713494924451));
#33888=CARTESIAN_POINT('Ctrl Pts',(0.37459107121508,0.178707793242271,-0.422930059276854));
#33889=CARTESIAN_POINT('Ctrl Pts',(0.0572948166238478,0.411062343188925,
-0.411146623629255));
#33890=CARTESIAN_POINT('Ctrl Pts',(-0.278444336628561,0.28656647445625,
-0.400417777271984));
#33891=CARTESIAN_POINT('Ctrl Pts',(-0.351536125378526,0.0845672608314457,
-0.393616742797245));
#33892=CARTESIAN_POINT('Ctrl Pts',(-0.352256412867894,-0.000300619911437438,
-0.390743520205039));
#33893=CARTESIAN_POINT('Ctrl Pts',(-0.352250282015284,-0.000300002405069236,
-0.450956479794959));
#33894=CARTESIAN_POINT('Ctrl Pts',(-0.35251557432598,-0.0316694991392887,
-0.449894504732885));
#33895=CARTESIAN_POINT('Ctrl Pts',(-0.334412778538798,-0.178761099283432,
-0.444904717788278));
#33896=CARTESIAN_POINT('Ctrl Pts',(-0.129265949902175,-0.394392231601152,
-0.435987118961139));
#33897=CARTESIAN_POINT('Ctrl Pts',(0.257874911974541,-0.325200627191768,
-0.42420368331354));
#33898=CARTESIAN_POINT('Ctrl Pts',(0.413473132937555,0.0359845312630004,
-0.412420247665942));
#33899=CARTESIAN_POINT('Ctrl Pts',(0.197819026895949,0.364859631570464,
-0.400636812018343));
#33900=CARTESIAN_POINT('Ctrl Pts',(-0.195454295996888,0.366131856477703,
-0.388853376370746));
#33901=CARTESIAN_POINT('Ctrl Pts',(-0.347498740933083,0.137501831020397,
-0.38062659896295));
#33902=CARTESIAN_POINT('Ctrl Pts',(-0.352872465670038,0.0110992473866874,
-0.376327633437688));
#33903=CARTESIAN_POINT('Ctrl Pts',(-0.352803593413643,0.000180282396865497,
-0.375956479794959));
#33904=CARTESIAN_POINT('Origin',(0.,0.,-0.953243520205039));
#33905=CARTESIAN_POINT('',(-0.352926766978824,3.65888010280694E-6,-0.54074352020504));
#33906=CARTESIAN_POINT('',(-0.351984139032922,0.000221539830159989,-0.52595647979496));
#33907=CARTESIAN_POINT('',(-0.352375,-1.84016574122319E-14,-0.953243520205039));
#33908=CARTESIAN_POINT('Ctrl Pts',(-0.352926747396533,3.65875024863191E-6,
-0.54074352020504));
#33909=CARTESIAN_POINT('Ctrl Pts',(-0.352908681542431,-0.115236454325059,
-0.536822673505106));
#33910=CARTESIAN_POINT('Ctrl Pts',(-0.229082675555813,-0.345954773140889,
-0.528974014922639));
#33911=CARTESIAN_POINT('Ctrl Pts',(0.162305420542359,-0.381984157190963,
-0.517197544457641));
#33912=CARTESIAN_POINT('Ctrl Pts',(0.408193007052407,-0.0750560794736075,
-0.505414108810041));
#33913=CARTESIAN_POINT('Ctrl Pts',(0.287569224913323,0.299263908404139,
-0.493630673162444));
#33914=CARTESIAN_POINT('Ctrl Pts',(-0.09125934819834,0.40487859581871,-0.481847237514845));
#33915=CARTESIAN_POINT('Ctrl Pts',(-0.32546833938393,0.201410083407456,
-0.472551519862377));
#33916=CARTESIAN_POINT('Ctrl Pts',(-0.352228200276193,0.0428406751097234,
-0.467183614092442));
#33917=CARTESIAN_POINT('Ctrl Pts',(-0.351979915865352,0.000219139502586143,
-0.46574352020504));
#33918=CARTESIAN_POINT('Ctrl Pts',(-0.351984139032922,0.000221539830159961,
-0.52595647979496));
#33919=CARTESIAN_POINT('Ctrl Pts',(-0.351548904827268,-0.0736221937851192,
-0.523461376028082));
#33920=CARTESIAN_POINT('Ctrl Pts',(-0.293017054148803,-0.264342833231124,
-0.517038460378671));
#33921=CARTESIAN_POINT('Ctrl Pts',(0.0180311431761832,-0.414644180006055,
-0.506687732846728));
#33922=CARTESIAN_POINT('Ctrl Pts',(0.355943505618862,-0.213445868946458,
-0.49490429719913));
#33923=CARTESIAN_POINT('Ctrl Pts',(0.374258670005346,0.17940280397765,-0.483120861551532));
#33924=CARTESIAN_POINT('Ctrl Pts',(0.0565316805849977,0.411167955025903,
-0.471337425903933));
#33925=CARTESIAN_POINT('Ctrl Pts',(-0.278744807800919,0.286135228707803,
-0.460615965318409));
#33926=CARTESIAN_POINT('Ctrl Pts',(-0.35153436645443,0.0843534532086563,
-0.453822316615418));
#33927=CARTESIAN_POINT('Ctrl Pts',(-0.352250282015284,-0.000300002405069236,
-0.450956479794959));
#33928=CARTESIAN_POINT('Origin',(0.,0.,-0.953243520205039));
#33929=CARTESIAN_POINT('',(-0.351987971037649,-0.000223646241047472,-0.61574352020504));
#33930=CARTESIAN_POINT('',(-0.35292677092685,-2.20166561067338E-7,-0.60095647979496));
#33931=CARTESIAN_POINT('',(-0.352375,-1.84016574122319E-14,-0.953243520205039));
#33932=CARTESIAN_POINT('Ctrl Pts',(-0.351987971037649,-0.000223646241047443,
-0.61574352020504));
#33933=CARTESIAN_POINT('Ctrl Pts',(-0.352239290406269,-0.0424304558714861,
-0.614317356682835));
#33934=CARTESIAN_POINT('Ctrl Pts',(-0.325821604001666,-0.200575489607239,
-0.608963381278098));
#33935=CARTESIAN_POINT('Ctrl Pts',(-0.0926762852132086,-0.404556616836208,
-0.599681593990828));
#33936=CARTESIAN_POINT('Ctrl Pts',(0.286519709527895,-0.300268871483724,
-0.58789815834323));
#33937=CARTESIAN_POINT('Ctrl Pts',(0.408453286141698,0.0736265026253448,
-0.576114722695632));
#33938=CARTESIAN_POINT('Ctrl Pts',(0.163641779290076,0.381413573840065,
-0.564331287048033));
#33939=CARTESIAN_POINT('Ctrl Pts',(-0.228101616324409,0.34673418884258,
-0.552547851400434));
#33940=CARTESIAN_POINT('Ctrl Pts',(-0.352834663655244,0.115857896512362,
-0.544685262452771));
#33941=CARTESIAN_POINT('Ctrl Pts',(-0.352926779489594,0.000208376886847085,
-0.540750485387639));
#33942=CARTESIAN_POINT('Ctrl Pts',(-0.352926747396533,3.65875024863191E-6,
-0.54074352020504));
#33943=CARTESIAN_POINT('Ctrl Pts',(-0.352926770854712,-2.20166532327402E-7,
-0.60095647979496));
#33944=CARTESIAN_POINT('Ctrl Pts',(-0.352926770972352,-1.2581965258919E-5,
-0.600956059205812));
#33945=CARTESIAN_POINT('Ctrl Pts',(-0.352921218665278,-0.115469719509711,
-0.597027826734131));
#33946=CARTESIAN_POINT('Ctrl Pts',(-0.22867160906457,-0.346358504439924,
-0.589171782379916));
#33947=CARTESIAN_POINT('Ctrl Pts',(0.163014183448326,-0.38168218876817,
-0.577388346732319));
#33948=CARTESIAN_POINT('Ctrl Pts',(0.408331593749854,-0.0742982379650506,
-0.56560491108472));
#33949=CARTESIAN_POINT('Ctrl Pts',(0.28701319867986,0.299797167962814,-0.553821475437122));
#33950=CARTESIAN_POINT('Ctrl Pts',(-0.0920107376299498,0.404708465680984,
-0.542038039789523));
#33951=CARTESIAN_POINT('Ctrl Pts',(-0.325655832183524,0.200967578910638,
-0.532749707908803));
#33952=CARTESIAN_POINT('Ctrl Pts',(-0.352234053921003,0.0426231897516333,
-0.527389187910615));
#33953=CARTESIAN_POINT('Ctrl Pts',(-0.351984139032922,0.000221539830159961,
-0.52595647979496));
#33954=CARTESIAN_POINT('Origin',(0.,0.,-0.953243520205039));
#33955=CARTESIAN_POINT('',(-0.352244141620507,0.000298967984602608,-0.69074352020504));
#33956=CARTESIAN_POINT('',(-0.351983621638971,-0.000221293924554444,-0.67595647979496));
#33957=CARTESIAN_POINT('',(-0.352375,-1.84016574122319E-14,-0.953243520205039));
#33958=CARTESIAN_POINT('Ctrl Pts',(-0.352244141620507,0.000298967984602598,
-0.69074352020504));
#33959=CARTESIAN_POINT('Ctrl Pts',(-0.351532316544511,-0.0841643753389943,
-0.687884227978032));
#33960=CARTESIAN_POINT('Ctrl Pts',(-0.279011704689758,-0.285752370658725,
-0.681097123868492));
#33961=CARTESIAN_POINT('Ctrl Pts',(0.055855997335481,-0.411260820487245,
-0.670382207876418));
#33962=CARTESIAN_POINT('Ctrl Pts',(0.373962743705146,-0.180017958610726,
-0.65859877222882));
#33963=CARTESIAN_POINT('Ctrl Pts',(0.356294325733907,0.212860018649936,
-0.646815336581221));
#33964=CARTESIAN_POINT('Ctrl Pts',(0.0187130423499051,0.414614052167785,
-0.635031900933623));
#33965=CARTESIAN_POINT('Ctrl Pts',(-0.292778674157529,0.264729732699978,
-0.624674628808229));
#33966=CARTESIAN_POINT('Ctrl Pts',(-0.351547129102879,0.0738117602623278,
-0.618245168565368));
#33967=CARTESIAN_POINT('Ctrl Pts',(-0.351987971037649,-0.000223646241047443,
-0.61574352020504));
#33968=CARTESIAN_POINT('Ctrl Pts',(-0.351983621638971,-0.000221293924554434,
-0.67595647979496));
#33969=CARTESIAN_POINT('Ctrl Pts',(-0.352233383192499,-0.0426479614893011,
-0.674522930501008));
#33970=CARTESIAN_POINT('Ctrl Pts',(-0.325634615254823,-0.201017878084083,
-0.669161569324524));
#33971=CARTESIAN_POINT('Ctrl Pts',(-0.0919250879749927,-0.404727983568883,
-0.659872396265506));
#33972=CARTESIAN_POINT('Ctrl Pts',(0.287076527003714,-0.299736444131386,
-0.64808896061791));
#33973=CARTESIAN_POINT('Ctrl Pts',(0.408315900728571,0.074384541261718,
-0.636305524970309));
#33974=CARTESIAN_POINT('Ctrl Pts',(0.162933476272259,0.381716654782934,
-0.624522089322712));
#33975=CARTESIAN_POINT('Ctrl Pts',(-0.228730842945548,0.346311409591309,
-0.612739074264261));
#33976=CARTESIAN_POINT('Ctrl Pts',(-0.352925672358273,0.115432193888956,
-0.604883871088345));
#33977=CARTESIAN_POINT('Ctrl Pts',(-0.352926770854712,-2.20166532327402E-7,
-0.60095647979496));
#33978=CARTESIAN_POINT('Origin',(0.,0.,-0.953243520205039));
#33979=CARTESIAN_POINT('',(-0.352786263833399,-0.000190149253296143,-0.76574352020504));
#33980=CARTESIAN_POINT('',(-0.352246168648578,0.000295985828685064,-0.75095647979496));
#33981=CARTESIAN_POINT('',(-0.352375,-1.84016574122319E-14,-0.953243520205039));
#33982=CARTESIAN_POINT('Ctrl Pts',(-0.352786263833399,-0.000190149253296124,
-0.76574352020504));
#33983=CARTESIAN_POINT('Ctrl Pts',(-0.352849014341479,-0.0109186220279966,
-0.765378911155762));
#33984=CARTESIAN_POINT('Ctrl Pts',(-0.347537096564293,-0.137150916764344,
-0.761086490223951));
#33985=CARTESIAN_POINT('Ctrl Pts',(-0.196120693160165,-0.365772397335523,
-0.752866257409607));
#33986=CARTESIAN_POINT('Ctrl Pts',(0.197252328460035,-0.365204165813244,
-0.741082821762008));
#33987=CARTESIAN_POINT('Ctrl Pts',(0.413395790837222,-0.036654313951176,
-0.72929938611441));
#33988=CARTESIAN_POINT('Ctrl Pts',(0.258418710730661,0.324770678736576,
-0.717515950466812));
#33989=CARTESIAN_POINT('Ctrl Pts',(-0.128621903482862,0.394607163242637,
-0.705732514819214));
#33990=CARTESIAN_POINT('Ctrl Pts',(-0.334268395112202,0.179152490472527,
-0.696808371398623));
#33991=CARTESIAN_POINT('Ctrl Pts',(-0.352510151186726,0.0318629829041549,
-0.691812039860565));
#33992=CARTESIAN_POINT('Ctrl Pts',(-0.352244141620507,0.000298967984602598,
-0.69074352020504));
#33993=CARTESIAN_POINT('Ctrl Pts',(-0.352246168648579,0.000295985828685053,
-0.75095647979496));
#33994=CARTESIAN_POINT('Ctrl Pts',(-0.351530728592248,-0.0843810609727061,
-0.748089801796205));
#33995=CARTESIAN_POINT('Ctrl Pts',(-0.278717649207867,-0.286178366077153,
-0.741295311914916));
#33996=CARTESIAN_POINT('Ctrl Pts',(0.056622872027267,-0.411159623934646,
-0.730573010151098));
#33997=CARTESIAN_POINT('Ctrl Pts',(0.374294355448138,-0.179321777388505,
-0.718789574503498));
#33998=CARTESIAN_POINT('Ctrl Pts',(0.355899542327467,0.213520119856154,
-0.7070061388559));
#33999=CARTESIAN_POINT('Ctrl Pts',(0.017942870124783,0.414648503505772,
-0.695222703208303));
#34000=CARTESIAN_POINT('Ctrl Pts',(-0.29304745006662,0.26429292408189,-0.684872816854654));
#34001=CARTESIAN_POINT('Ctrl Pts',(-0.351549056255237,0.0735977579290679,
-0.678450742383541));
#34002=CARTESIAN_POINT('Ctrl Pts',(-0.351983621638971,-0.000221293924554434,
-0.67595647979496));
#34003=CARTESIAN_POINT('Ctrl Pts',(-0.350836093496678,-0.0328964454765271,
-0.824840495331884));
#34004=CARTESIAN_POINT('Ctrl Pts',(-0.340011333932142,-0.148341026301304,
-0.820912683449351));
#34005=CARTESIAN_POINT('Ctrl Pts',(-0.195816346135933,-0.365812208923844,
-0.813057059684284));
#34006=CARTESIAN_POINT('Ctrl Pts',(0.198108374437807,-0.364996837653778,
-0.801273624036688));
#34007=CARTESIAN_POINT('Ctrl Pts',(0.413371658758658,-0.0358045106953606,
-0.789490188389087));
#34008=CARTESIAN_POINT('Ctrl Pts',(0.257863027527083,0.32520678286678,-0.777706752741491));
#34009=CARTESIAN_POINT('Ctrl Pts',(-0.129379073725142,0.394390194728457,
-0.765923317093891));
#34010=CARTESIAN_POINT('Ctrl Pts',(-0.400348103178378,0.109366128011736,
-0.754139881446294));
#34011=CARTESIAN_POINT('Ctrl Pts',(-0.311904664228006,-0.273809580860039,
-0.742356445798694));
#34012=CARTESIAN_POINT('Ctrl Pts',(0.056622872027267,-0.411159623934646,
-0.730573010151098));
#34013=CARTESIAN_POINT('Ctrl Pts',(0.374294355448138,-0.179321777388505,
-0.718789574503498));
#34014=CARTESIAN_POINT('Ctrl Pts',(0.355899542327467,0.213520119856154,
-0.7070061388559));
#34015=CARTESIAN_POINT('Ctrl Pts',(0.017942870124783,0.414648503505772,
-0.695222703208303));
#34016=CARTESIAN_POINT('Ctrl Pts',(-0.336122314727238,0.243467368383994,
-0.683439267560703));
#34017=CARTESIAN_POINT('Ctrl Pts',(-0.38838863294677,-0.146319091464592,
-0.671655831913106));
#34018=CARTESIAN_POINT('Ctrl Pts',(-0.0919250879749927,-0.404727983568883,
-0.659872396265506));
#34019=CARTESIAN_POINT('Ctrl Pts',(0.287076527003714,-0.299736444131386,
-0.64808896061791));
#34020=CARTESIAN_POINT('Ctrl Pts',(0.408315900728571,0.074384541261718,
-0.636305524970309));
#34021=CARTESIAN_POINT('Ctrl Pts',(0.162933476272259,0.381716654782934,
-0.624522089322712));
#34022=CARTESIAN_POINT('Ctrl Pts',(-0.22874482321813,0.346310145817832,
-0.612738653675113));
#34023=CARTESIAN_POINT('Ctrl Pts',(-0.4150360455362,-4.38686883980485E-5,
-0.600955218027516));
#34024=CARTESIAN_POINT('Ctrl Pts',(-0.22867160906457,-0.346358504439924,
-0.589171782379916));
#34025=CARTESIAN_POINT('Ctrl Pts',(0.163014183448326,-0.38168218876817,
-0.577388346732319));
#34026=CARTESIAN_POINT('Ctrl Pts',(0.408331593749854,-0.0742982379650506,
-0.56560491108472));
#34027=CARTESIAN_POINT('Ctrl Pts',(0.28701319867986,0.299797167962814,-0.553821475437122));
#34028=CARTESIAN_POINT('Ctrl Pts',(-0.0920107376299498,0.404708465680984,
-0.542038039789523));
#34029=CARTESIAN_POINT('Ctrl Pts',(-0.38841939005586,0.14623712132408,-0.530254604141926));
#34030=CARTESIAN_POINT('Ctrl Pts',(-0.336071155929779,-0.243538695681005,
-0.518471168494327));
#34031=CARTESIAN_POINT('Ctrl Pts',(0.0180311431761832,-0.414644180006055,
-0.506687732846728));
#34032=CARTESIAN_POINT('Ctrl Pts',(0.355943505618862,-0.213445868946458,
-0.49490429719913));
#34033=CARTESIAN_POINT('Ctrl Pts',(0.374258670005346,0.17940280397765,-0.483120861551532));
#34034=CARTESIAN_POINT('Ctrl Pts',(0.0565316805849977,0.411167955025903,
-0.471337425903933));
#34035=CARTESIAN_POINT('Ctrl Pts',(-0.311954394006589,0.273750569338514,
-0.459553990256335));
#34036=CARTESIAN_POINT('Ctrl Pts',(-0.400340540765316,-0.109464010390782,
-0.447770554608737));
#34037=CARTESIAN_POINT('Ctrl Pts',(-0.129265949902175,-0.394392231601152,
-0.435987118961139));
#34038=CARTESIAN_POINT('Ctrl Pts',(0.257874911974541,-0.325200627191768,
-0.42420368331354));
#34039=CARTESIAN_POINT('Ctrl Pts',(0.413473132937555,0.0359845312630004,
-0.412420247665942));
#34040=CARTESIAN_POINT('Ctrl Pts',(0.197819026895949,0.364859631570464,
-0.400636812018343));
#34041=CARTESIAN_POINT('Ctrl Pts',(-0.195454295996888,0.366131856477703,
-0.388853376370746));
#34042=CARTESIAN_POINT('Ctrl Pts',(-0.413231664177891,0.0386588912395302,
-0.377069940723146));
#34043=CARTESIAN_POINT('Ctrl Pts',(-0.259973517118929,-0.323525406343912,
-0.365286505075549));
#34044=CARTESIAN_POINT('Ctrl Pts',(0.126711582028227,-0.395220309612058,
-0.353503069427949));
#34045=CARTESIAN_POINT('Ctrl Pts',(0.399623944950114,-0.112051866435688,
-0.341719633780353));
#34046=CARTESIAN_POINT('Ctrl Pts',(0.313718992635124,0.271726538679157,
-0.329936198132753));
#34047=CARTESIAN_POINT('Ctrl Pts',(-0.0538702984580581,0.411525101398655,
-0.318152762485156));
#34048=CARTESIAN_POINT('Ctrl Pts',(-0.373090125879399,0.181820450206457,
-0.306369326837557));
#34049=CARTESIAN_POINT('Ctrl Pts',(-0.357317020662606,-0.211138497127641,
-0.294585891189959));
#34050=CARTESIAN_POINT('Ctrl Pts',(-0.0207134553279411,-0.414518842516768,
-0.28280245554236));
#34051=CARTESIAN_POINT('Ctrl Pts',(0.334488460689772,-0.245707931903623,
-0.271019019894762));
#34052=CARTESIAN_POINT('Ctrl Pts',(0.389357394519836,0.14372104213278,-0.259235584247163));
#34053=CARTESIAN_POINT('Ctrl Pts',(0.0946272181670758,0.404104697832314,
-0.247452148599565));
#34054=CARTESIAN_POINT('Ctrl Pts',(-0.285067544718883,0.301647829990517,
-0.235668712951967));
#34055=CARTESIAN_POINT('Ctrl Pts',(-0.408803749032928,-0.0716548379065293,
-0.223885277304369));
#34056=CARTESIAN_POINT('Ctrl Pts',(-0.16548019720029,-0.380619515500736,
-0.21210184165677));
#34057=CARTESIAN_POINT('Ctrl Pts',(0.226425923378982,-0.347830739657686,
-0.200318406009172));
#34058=CARTESIAN_POINT('Ctrl Pts',(0.415027091810056,-0.00272907130485191,
-0.188534970361573));
#34059=CARTESIAN_POINT('Ctrl Pts',(0.230980581763497,0.344822909832333,
-0.176751534713975));
#34060=CARTESIAN_POINT('Ctrl Pts',(-0.160460352000493,0.382762900395039,
-0.164968099066377));
#34061=CARTESIAN_POINT('Ctrl Pts',(-0.40782621365004,0.0770245817201009,
-0.153184663418778));
#34062=CARTESIAN_POINT('Ctrl Pts',(-0.289009548904106,-0.29787254080843,
-0.14140122777118));
#34063=CARTESIAN_POINT('Ctrl Pts',(0.0893042060071663,-0.40531479967714,
-0.129617792123582));
#34064=CARTESIAN_POINT('Ctrl Pts',(0.387434651449787,-0.148827808786758,
-0.117834356475983));
#34065=CARTESIAN_POINT('Ctrl Pts',(0.33768892962625,0.241285621564956,-0.106050920828385));
#34066=CARTESIAN_POINT('Ctrl Pts',(-0.0152568165427812,0.414759708192197,
-0.0942674851807867));
#34067=CARTESIAN_POINT('Ctrl Pts',(-0.354516303198198,0.215811021276995,
-0.0824840495331884));
#34068=CARTESIAN_POINT('Ctrl Pts',(-0.375435905852211,-0.176882543716822,
-0.07070061388559));
#34069=CARTESIAN_POINT('Ctrl Pts',(-0.0593024712652474,-0.410811133390711,
-0.0589171782379917));
#34070=CARTESIAN_POINT('Ctrl Pts',(0.31016609475332,-0.275771257119863,
-0.0471337425903933));
#34071=CARTESIAN_POINT('Ctrl Pts',(0.400971528752744,0.106676728393338,
-0.0353503069427951));
#34072=CARTESIAN_POINT('Ctrl Pts',(0.13207620156309,0.39373277295688,-0.0235668712951966));
#34073=CARTESIAN_POINT('Ctrl Pts',(-0.256066899639439,0.326484848838067,
-0.0117834356475983));
#34074=CARTESIAN_POINT('Ctrl Pts',(-0.360525536959465,0.0873733625685078,
-0.00392781188253277));
#34075=CARTESIAN_POINT('Ctrl Pts',(-0.351244341336214,-0.0282055544935645,
0.));
#34076=CARTESIAN_POINT('Ctrl Pts',(-0.365115126650463,-0.0342353311964058,
-0.816560330221256));
#34077=CARTESIAN_POINT('Ctrl Pts',(-0.353849799243652,-0.154378507825829,
-0.812632518338723));
#34078=CARTESIAN_POINT('Ctrl Pts',(-0.203786073739102,-0.3807007701526,
-0.804776894573657));
#34079=CARTESIAN_POINT('Ctrl Pts',(0.206171387619962,-0.3798522132622,-0.792993458926059));
#34080=CARTESIAN_POINT('Ctrl Pts',(0.430195890158058,-0.0372617547040343,
-0.781210023278461));
#34081=CARTESIAN_POINT('Ctrl Pts',(0.268358055796544,0.338442702774873,
-0.769426587630862));
#34082=CARTESIAN_POINT('Ctrl Pts',(-0.134644803555601,0.410441880317382,
-0.757643151983264));
#34083=CARTESIAN_POINT('Ctrl Pts',(-0.416642275711663,0.113817330715017,
-0.745859716335666));
#34084=CARTESIAN_POINT('Ctrl Pts',(-0.324599187750211,-0.28495363403871,
-0.734076280688068));
#34085=CARTESIAN_POINT('Ctrl Pts',(0.0589274235883146,-0.427893825490553,
-0.722292845040469));
#34086=CARTESIAN_POINT('Ctrl Pts',(0.389528140140729,-0.186620175848612,
-0.710509409392871));
#34087=CARTESIAN_POINT('Ctrl Pts',(0.370384657908538,0.222210391259072,
-0.698725973745272));
#34088=CARTESIAN_POINT('Ctrl Pts',(0.0186731451510285,0.431524702501478,
-0.686942538097674));
#34089=CARTESIAN_POINT('Ctrl Pts',(-0.349802496911123,0.253376493156109,
-0.675159102450075));
#34090=CARTESIAN_POINT('Ctrl Pts',(-0.404196054900214,-0.152274280217354,
-0.663375666802478));
#34091=CARTESIAN_POINT('Ctrl Pts',(-0.0956664401425461,-0.421200417285852,
-0.65159223115488));
#34092=CARTESIAN_POINT('Ctrl Pts',(0.298760545047307,-0.311935720951775,
-0.639808795507281));
#34093=CARTESIAN_POINT('Ctrl Pts',(0.424934362716365,0.0774119929706307,
-0.628025359859682));
#34094=CARTESIAN_POINT('Ctrl Pts',(0.169564870683152,0.397252527146217,
-0.616241924212084));
#34095=CARTESIAN_POINT('Ctrl Pts',(-0.238054740227906,0.36040497284757,
-0.604458488564485));
#34096=CARTESIAN_POINT('Ctrl Pts',(-0.431928017497127,-4.56541445331377E-5,
-0.592675052916888));
#34097=CARTESIAN_POINT('Ctrl Pts',(-0.237978546257431,-0.360455299666153,
-0.580891617269288));
#34098=CARTESIAN_POINT('Ctrl Pts',(0.169648862642238,-0.397216658364245,
-0.569108181621692));
#34099=CARTESIAN_POINT('Ctrl Pts',(0.4249506944438,-0.0773221771287707,
-0.557324745974091));
#34100=CARTESIAN_POINT('Ctrl Pts',(0.298694639259925,0.311998916243858,
-0.545541310326495));
#34101=CARTESIAN_POINT('Ctrl Pts',(-0.0957555757394711,0.421180105019685,
-0.533757874678895));
#34102=CARTESIAN_POINT('Ctrl Pts',(-0.404228063824008,0.152188973891156,
-0.521974439031298));
#34103=CARTESIAN_POINT('Ctrl Pts',(-0.349749255950003,-0.25345072347495,
-0.510191003383699));
#34104=CARTESIAN_POINT('Ctrl Pts',(0.0187650109166624,-0.431520203035271,
-0.498407567736101));
#34105=CARTESIAN_POINT('Ctrl Pts',(0.370430410506412,-0.222133118336476,
-0.486624132088503));
#34106=CARTESIAN_POINT('Ctrl Pts',(0.389491002299994,0.186704500220892,
-0.474840696440904));
#34107=CARTESIAN_POINT('Ctrl Pts',(0.0588325206532684,0.427902495657323,
-0.463057260793306));
#34108=CARTESIAN_POINT('Ctrl Pts',(-0.324650941531368,0.284892220747562,
-0.451273825145707));
#34109=CARTESIAN_POINT('Ctrl Pts',(-0.4166344055083,-0.113919196908045,
-0.439490389498109));
#34110=CARTESIAN_POINT('Ctrl Pts',(-0.134527075591703,-0.41044400009082,
-0.42770695385051));
#34111=CARTESIAN_POINT('Ctrl Pts',(0.268370423941152,-0.338436296563816,
-0.415923518202913));
#34112=CARTESIAN_POINT('Ctrl Pts',(0.430301494337237,0.0374491021109036,
-0.404140082555314));
#34113=CARTESIAN_POINT('Ctrl Pts',(0.205870263629731,0.379709422889672,
-0.392356646907716));
#34114=CARTESIAN_POINT('Ctrl Pts',(-0.203409288155115,0.381033427365681,
-0.380573211260117));
#34115=CARTESIAN_POINT('Ctrl Pts',(-0.430050197796199,0.0402323085701024,
-0.368789775612519));
#34116=CARTESIAN_POINT('Ctrl Pts',(-0.270554442339733,-0.336692894207642,
-0.357006339964921));
#34117=CARTESIAN_POINT('Ctrl Pts',(0.13186874491508,-0.411305780886562,
-0.345222904317323));
#34118=CARTESIAN_POINT('Ctrl Pts',(0.415888644234946,-0.116612378724581,
-0.333439468669723));
#34119=CARTESIAN_POINT('Ctrl Pts',(0.326487359344952,0.282785812016435,
-0.321656033022126));
#34120=CARTESIAN_POINT('Ctrl Pts',(-0.056062820242291,0.428274177891669,
-0.309872597374527));
#34121=CARTESIAN_POINT('Ctrl Pts',(-0.388274898414303,0.1892205446798,-0.298089161726929));
#34122=CARTESIAN_POINT('Ctrl Pts',(-0.371859827628678,-0.219731836457348,
-0.286305726079331));
#34123=CARTESIAN_POINT('Ctrl Pts',(-0.021556493204716,-0.431389764308688,
-0.274522290431732));
#34124=CARTESIAN_POINT('Ctrl Pts',(0.348102144995012,-0.255708247637481,
-0.262738854784134));
#34125=CARTESIAN_POINT('Ctrl Pts',(0.40520424508076,0.149570490247016,-0.250955419136536));
#34126=CARTESIAN_POINT('Ctrl Pts',(0.0984785470653985,0.420551763812434,
-0.239171983488937));
#34127=CARTESIAN_POINT('Ctrl Pts',(-0.296669797159729,0.313924900237974,
-0.227388547841339));
#34128=CARTESIAN_POINT('Ctrl Pts',(-0.425442066452478,-0.0745711906566084,
-0.215605112193741));
#34129=CARTESIAN_POINT('Ctrl Pts',(-0.172215243183067,-0.396110734282261,
-0.203821676546142));
#34130=CARTESIAN_POINT('Ctrl Pts',(0.235641461137884,-0.361987454874687,
-0.192038240898544));
#34131=CARTESIAN_POINT('Ctrl Pts',(0.431918699354223,-0.00284014453923051,
-0.180254805250946));
#34132=CARTESIAN_POINT('Ctrl Pts',(0.240381494172507,0.358857206339876,
-0.168471369603347));
#34133=CARTESIAN_POINT('Ctrl Pts',(-0.166991090224279,0.398341354967106,
-0.156687933955749));
#34134=CARTESIAN_POINT('Ctrl Pts',(-0.424424745367948,0.0801594831068888,
-0.14490449830815));
#34135=CARTESIAN_POINT('Ctrl Pts',(-0.300772240961904,-0.309995956741533,
-0.133121062660552));
#34136=CARTESIAN_POINT('Ctrl Pts',(0.0929388882476368,-0.421811116816654,
-0.121337627012954));
#34137=CARTESIAN_POINT('Ctrl Pts',(0.403203246345024,-0.154885102364198,
-0.109554191365355));
#34138=CARTESIAN_POINT('Ctrl Pts',(0.351432873055049,0.251105949215736,
-0.0977707557177572));
#34139=CARTESIAN_POINT('Ctrl Pts',(-0.015877769156476,0.431640433219955,
-0.0859873200701588));
#34140=CARTESIAN_POINT('Ctrl Pts',(-0.368945120930351,0.224594532394832,
-0.0742038844225605));
#34141=CARTESIAN_POINT('Ctrl Pts',(-0.390716151659747,-0.184081665337648,
-0.0624204487749621));
#34142=CARTESIAN_POINT('Ctrl Pts',(-0.0617160825469674,-0.427531151377359,
-0.0506370131273638));
#34143=CARTESIAN_POINT('Ctrl Pts',(0.322789858477346,-0.286995150545506,
-0.0388535774797655));
#34144=CARTESIAN_POINT('Ctrl Pts',(0.417291074714279,0.111018472500347,
-0.0270701418321671));
#34145=CARTESIAN_POINT('Ctrl Pts',(0.137451704528447,0.409757701471928,
-0.0152867061845688));
#34146=CARTESIAN_POINT('Ctrl Pts',(-0.266488825482632,0.339772786046305,
-0.0035032705369704));
#34147=CARTESIAN_POINT('Ctrl Pts',(-0.375198930576758,0.0909294594581953,
0.00435235322809514));
#34148=CARTESIAN_POINT('Ctrl Pts',(-0.365539990181895,-0.0293535208949691,
0.0082801651106279));
#34149=CARTESIAN_POINT('Ctrl Pts',(-0.379394159804248,-0.0355742169162846,
-0.808280165110628));
#34150=CARTESIAN_POINT('Ctrl Pts',(-0.367688264555163,-0.160415989350353,
-0.804352353228095));
#34151=CARTESIAN_POINT('Ctrl Pts',(-0.21175580134227,-0.395589331381355,
-0.79649672946303));
#34152=CARTESIAN_POINT('Ctrl Pts',(0.214234400802117,-0.394707588870624,
-0.784713293815431));
#34153=CARTESIAN_POINT('Ctrl Pts',(0.447020121557459,-0.0387189987127072,
-0.772929858167834));
#34154=CARTESIAN_POINT('Ctrl Pts',(0.278853084066004,0.351678622682965,
-0.761146422520234));
#34155=CARTESIAN_POINT('Ctrl Pts',(-0.13991053338606,0.426493565906307,
-0.749362986872636));
#34156=CARTESIAN_POINT('Ctrl Pts',(-0.432936448244949,0.118268533418297,
-0.737579551225038));
#34157=CARTESIAN_POINT('Ctrl Pts',(-0.337293711272416,-0.29609768721738,
-0.72579611557744));
#34158=CARTESIAN_POINT('Ctrl Pts',(0.0612319751493615,-0.44462802704646,
-0.71401267992984));
#34159=CARTESIAN_POINT('Ctrl Pts',(0.404761924833321,-0.193918574308719,
-0.702229244282244));
#34160=CARTESIAN_POINT('Ctrl Pts',(0.384869773489609,0.230900662661991,
-0.690445808634644));
#34161=CARTESIAN_POINT('Ctrl Pts',(0.0194034201772741,0.448400901497184,
-0.678662372987047));
#34162=CARTESIAN_POINT('Ctrl Pts',(-0.363482679095007,0.263285617928224,
-0.666878937339448));
#34163=CARTESIAN_POINT('Ctrl Pts',(-0.420003476853659,-0.158229468970116,
-0.65509550169185));
#34164=CARTESIAN_POINT('Ctrl Pts',(-0.0994077923100996,-0.437672851002821,
-0.643312066044252));
#34165=CARTESIAN_POINT('Ctrl Pts',(0.310444563090901,-0.324134997772164,
-0.631528630396652));
#34166=CARTESIAN_POINT('Ctrl Pts',(0.441552824704159,0.0804394446795438,
-0.619745194749055));
#34167=CARTESIAN_POINT('Ctrl Pts',(0.176196265094044,0.4127883995095,-0.607961759101456));
#34168=CARTESIAN_POINT('Ctrl Pts',(-0.247364657237681,0.37449979987731,
-0.596178323453858));
#34169=CARTESIAN_POINT('Ctrl Pts',(-0.448819989458054,-4.74396006692321E-5,
-0.584394887806259));
#34170=CARTESIAN_POINT('Ctrl Pts',(-0.247285483450293,-0.374552094892382,
-0.572611452158662));
#34171=CARTESIAN_POINT('Ctrl Pts',(0.176283541836149,-0.41275112796032,
-0.560828016511063));
#34172=CARTESIAN_POINT('Ctrl Pts',(0.441569795137746,-0.0803461162924902,
-0.549044580863465));
#34173=CARTESIAN_POINT('Ctrl Pts',(0.310376079839991,0.324200664524903,
-0.537261145215866));
#34174=CARTESIAN_POINT('Ctrl Pts',(-0.0995004138489923,0.437651744358387,
-0.525477709568268));
#34175=CARTESIAN_POINT('Ctrl Pts',(-0.420036737592155,0.158140826458231,
-0.513694273920669));
#34176=CARTESIAN_POINT('Ctrl Pts',(-0.363427355970227,-0.263362751268896,
-0.501910838273072));
#34177=CARTESIAN_POINT('Ctrl Pts',(0.0194988786571419,-0.448396226064488,
-0.490127402625472));
#34178=CARTESIAN_POINT('Ctrl Pts',(0.384917315393962,-0.230820367726493,
-0.478343966977875));
#34179=CARTESIAN_POINT('Ctrl Pts',(0.404723334594643,0.194006196464134,
-0.466560531330276));
#34180=CARTESIAN_POINT('Ctrl Pts',(0.0611333607215388,0.444637036288742,
-0.454777095682678));
#34181=CARTESIAN_POINT('Ctrl Pts',(-0.337347489056148,0.296033872156611,
-0.442993660035079));
#34182=CARTESIAN_POINT('Ctrl Pts',(-0.432928270251285,-0.118374383425309,
-0.431210224387481));
#34183=CARTESIAN_POINT('Ctrl Pts',(-0.13978820128123,-0.426495768580487,
-0.419426788739883));
#34184=CARTESIAN_POINT('Ctrl Pts',(0.278865935907763,-0.351671965935864,
-0.407643353092284));
#34185=CARTESIAN_POINT('Ctrl Pts',(0.447129855736918,0.0389136729588066,
-0.395859917444686));
#34186=CARTESIAN_POINT('Ctrl Pts',(0.213921500363513,0.394559214208881,
-0.384076481797088));
#34187=CARTESIAN_POINT('Ctrl Pts',(-0.211364280313341,0.395934998253659,
-0.37229304614949));
#34188=CARTESIAN_POINT('Ctrl Pts',(-0.446868731414507,0.0418057259006754,
-0.360509610501891));
#34189=CARTESIAN_POINT('Ctrl Pts',(-0.281135367560537,-0.349860382071373,
-0.348726174854292));
#34190=CARTESIAN_POINT('Ctrl Pts',(0.137025907801932,-0.427391252161065,
-0.336942739206695));
#34191=CARTESIAN_POINT('Ctrl Pts',(0.432153343519779,-0.121172891013474,
-0.325159303559096));
#34192=CARTESIAN_POINT('Ctrl Pts',(0.33925572605478,0.293845085353713,-0.313375867911498));
#34193=CARTESIAN_POINT('Ctrl Pts',(-0.0582553420265235,0.445023254384683,
-0.301592432263899));
#34194=CARTESIAN_POINT('Ctrl Pts',(-0.403459670949207,0.196620639153144,
-0.289808996616301));
#34195=CARTESIAN_POINT('Ctrl Pts',(-0.386402634594751,-0.228325175787054,
-0.278025560968703));
#34196=CARTESIAN_POINT('Ctrl Pts',(-0.0223995310814905,-0.448260686100608,
-0.266242125321104));
#34197=CARTESIAN_POINT('Ctrl Pts',(0.361715829300251,-0.265708563371338,
-0.254458689673506));
#34198=CARTESIAN_POINT('Ctrl Pts',(0.421051095641684,0.155419938361253,
-0.242675254025907));
#34199=CARTESIAN_POINT('Ctrl Pts',(0.102329875963721,0.436998829792555,
-0.23089181837831));
#34200=CARTESIAN_POINT('Ctrl Pts',(-0.308272049600575,0.326201970485431,
-0.219108382730711));
#34201=CARTESIAN_POINT('Ctrl Pts',(-0.442080383872028,-0.077487543406688,
-0.207324947083113));
#34202=CARTESIAN_POINT('Ctrl Pts',(-0.178950289165844,-0.411601953063784,
-0.195541511435514));
#34203=CARTESIAN_POINT('Ctrl Pts',(0.244856998896787,-0.376144170091689,
-0.183758075787916));
#34204=CARTESIAN_POINT('Ctrl Pts',(0.44881030689839,-0.0029512177736084,
-0.171974640140318));
#34205=CARTESIAN_POINT('Ctrl Pts',(0.249782406581518,0.372891502847418,
-0.160191204492719));
#34206=CARTESIAN_POINT('Ctrl Pts',(-0.173521828448066,0.413919809539174,
-0.148407768845121));
#34207=CARTESIAN_POINT('Ctrl Pts',(-0.441023277085855,0.0832943844936766,
-0.136624333197523));
#34208=CARTESIAN_POINT('Ctrl Pts',(-0.312534933019702,-0.322119372674637,
-0.124840897549924));
#34209=CARTESIAN_POINT('Ctrl Pts',(0.0965735704881073,-0.438307433956169,
-0.113057461902326));
#34210=CARTESIAN_POINT('Ctrl Pts',(0.41897184124026,-0.160942395941638,
-0.101274026254728));
#34211=CARTESIAN_POINT('Ctrl Pts',(0.365176816483849,0.260926276866517,
-0.0894905906071292));
#34212=CARTESIAN_POINT('Ctrl Pts',(-0.016498721770171,0.448521158247713,
-0.0777071549595309));
#34213=CARTESIAN_POINT('Ctrl Pts',(-0.383373938662503,0.23337804351267,
-0.0659237193119325));
#34214=CARTESIAN_POINT('Ctrl Pts',(-0.405996397467284,-0.191280786958474,
-0.0541402836643343));
#34215=CARTESIAN_POINT('Ctrl Pts',(-0.0641296938286871,-0.444251169364007,
-0.0423568480167359));
#34216=CARTESIAN_POINT('Ctrl Pts',(0.335413622201372,-0.298219043971149,
-0.0305734123691375));
#34217=CARTESIAN_POINT('Ctrl Pts',(0.433610620675813,0.115360216607358,
-0.0187899767215392));
#34218=CARTESIAN_POINT('Ctrl Pts',(0.142827207493804,0.425782629986974,
-0.00700654107394083));
#34219=CARTESIAN_POINT('Ctrl Pts',(-0.276910751325826,0.353060723254543,
0.00477689457365749));
#34220=CARTESIAN_POINT('Ctrl Pts',(-0.389872324194051,0.0944855563478826,
0.012632518338723));
#34221=CARTESIAN_POINT('Ctrl Pts',(-0.379835639027576,-0.0305014872963737,
0.0165603302212558));
#34222=CARTESIAN_POINT('Ctrl Pts',(-0.393673192958032,-0.0369131026361633,
-0.8));
#34223=CARTESIAN_POINT('Ctrl Pts',(-0.381526729866674,-0.166453470874877,
-0.796072188117467));
#34224=CARTESIAN_POINT('Ctrl Pts',(-0.219725528945438,-0.410477892610111,
-0.788216564352402));
#34225=CARTESIAN_POINT('Ctrl Pts',(0.222297413984273,-0.409562964479047,
-0.776433128704804));
#34226=CARTESIAN_POINT('Ctrl Pts',(0.463844352956859,-0.0401762427213809,
-0.764649693057204));
#34227=CARTESIAN_POINT('Ctrl Pts',(0.289348112335464,0.364914542591059,
-0.752866257409607));
#34228=CARTESIAN_POINT('Ctrl Pts',(-0.145176263216518,0.442545251495232,
-0.741082821762008));
#34229=CARTESIAN_POINT('Ctrl Pts',(-0.449230620778234,0.122719736121578,
-0.72929938611441));
#34230=CARTESIAN_POINT('Ctrl Pts',(-0.349988234794621,-0.307241740396052,
-0.717515950466812));
#34231=CARTESIAN_POINT('Ctrl Pts',(0.0635365267104093,-0.461362228602367,
-0.705732514819213));
#34232=CARTESIAN_POINT('Ctrl Pts',(0.419995709525912,-0.201216972768827,
-0.693949079171616));
#34233=CARTESIAN_POINT('Ctrl Pts',(0.39935488907068,0.239590934064909,-0.682165643524016));
#34234=CARTESIAN_POINT('Ctrl Pts',(0.0201336952035193,0.465277100492891,
-0.670382207876419));
#34235=CARTESIAN_POINT('Ctrl Pts',(-0.377162861278892,0.273194742700339,
-0.658598772228819));
#34236=CARTESIAN_POINT('Ctrl Pts',(-0.435810898807103,-0.164184657722877,
-0.646815336581222));
#34237=CARTESIAN_POINT('Ctrl Pts',(-0.103149144477653,-0.454145284719791,
-0.635031900933623));
#34238=CARTESIAN_POINT('Ctrl Pts',(0.322128581134495,-0.336334274592552,
-0.623248465286026));
#34239=CARTESIAN_POINT('Ctrl Pts',(0.458171286691953,0.0834668963884565,
-0.611465029638426));
#34240=CARTESIAN_POINT('Ctrl Pts',(0.182827659504937,0.428324271872783,
-0.599681593990828));
#34241=CARTESIAN_POINT('Ctrl Pts',(-0.256674574247458,0.388594626907048,
-0.587898158343229));
#34242=CARTESIAN_POINT('Ctrl Pts',(-0.465711961418981,-4.92250568048239E-5,
-0.576114722695633));
#34243=CARTESIAN_POINT('Ctrl Pts',(-0.256592420643155,-0.388648890118611,
-0.564331287048032));
#34244=CARTESIAN_POINT('Ctrl Pts',(0.18291822103006,-0.428285597556395,
-0.552547851400436));
#34245=CARTESIAN_POINT('Ctrl Pts',(0.458188895831691,-0.0833700554562097,
-0.540764415752836));
#34246=CARTESIAN_POINT('Ctrl Pts',(0.322057520420056,0.336402412805948,
-0.528980980105239));
#34247=CARTESIAN_POINT('Ctrl Pts',(-0.103245251958514,0.454123383697088,
-0.51719754445764));
#34248=CARTESIAN_POINT('Ctrl Pts',(-0.435845411360303,0.164092679025306,
-0.505414108810041));
#34249=CARTESIAN_POINT('Ctrl Pts',(-0.377105455990451,-0.273274779062841,
-0.493630673162444));
#34250=CARTESIAN_POINT('Ctrl Pts',(0.0202327463976213,-0.465272249093704,
-0.481847237514844));
#34251=CARTESIAN_POINT('Ctrl Pts',(0.399404220281511,-0.23950761711651,
-0.470063801867247));
#34252=CARTESIAN_POINT('Ctrl Pts',(0.419955666889291,0.201307892707376,
-0.458280366219648));
#34253=CARTESIAN_POINT('Ctrl Pts',(0.0634342007898095,0.461371576920162,
-0.44649693057205));
#34254=CARTESIAN_POINT('Ctrl Pts',(-0.350044036580928,0.307175523565658,
-0.434713494924451));
#34255=CARTESIAN_POINT('Ctrl Pts',(-0.44922213499427,-0.122829569942572,
-0.422930059276853));
#34256=CARTESIAN_POINT('Ctrl Pts',(-0.145049326970758,-0.442547537070155,
-0.411146623629255));
#34257=CARTESIAN_POINT('Ctrl Pts',(0.289361447874374,-0.364907635307912,
-0.399363187981656));
#34258=CARTESIAN_POINT('Ctrl Pts',(0.4639582171366,0.0403782438067095,-0.387579752334058));
#34259=CARTESIAN_POINT('Ctrl Pts',(0.221972737097294,0.409409005528091,
-0.37579631668646));
#34260=CARTESIAN_POINT('Ctrl Pts',(-0.219319272471568,0.410836569141637,
-0.364012881038862));
#34261=CARTESIAN_POINT('Ctrl Pts',(-0.463687265032815,0.0433791432312484,
-0.352229445391263));
#34262=CARTESIAN_POINT('Ctrl Pts',(-0.291716292781341,-0.363027869935104,
-0.340446009743666));
#34263=CARTESIAN_POINT('Ctrl Pts',(0.142183070688784,-0.443476723435568,
-0.328662574096066));
#34264=CARTESIAN_POINT('Ctrl Pts',(0.448418042804611,-0.125733403302368,
-0.316879138448469));
#34265=CARTESIAN_POINT('Ctrl Pts',(0.352024092764608,0.304904358690991,
-0.305095702800869));
#34266=CARTESIAN_POINT('Ctrl Pts',(-0.0604478638107563,0.461772330877697,
-0.293312267153272));
#34267=CARTESIAN_POINT('Ctrl Pts',(-0.418644443484112,0.204020733626488,
-0.281528831505673));
#34268=CARTESIAN_POINT('Ctrl Pts',(-0.400945441560823,-0.236918515116761,
-0.269745395858075));
#34269=CARTESIAN_POINT('Ctrl Pts',(-0.0232425689582656,-0.465131607892529,
-0.257961960210476));
#34270=CARTESIAN_POINT('Ctrl Pts',(0.375329513605492,-0.275708879105196,
-0.246178524562878));
#34271=CARTESIAN_POINT('Ctrl Pts',(0.436897946202607,0.161269386475489,
-0.234395088915279));
#34272=CARTESIAN_POINT('Ctrl Pts',(0.106181204862043,0.453445895772676,
-0.222611653267682));
#34273=CARTESIAN_POINT('Ctrl Pts',(-0.31987430204142,0.338479040732887,
-0.210828217620083));
#34274=CARTESIAN_POINT('Ctrl Pts',(-0.458718701291578,-0.0804038961567671,
-0.199044781972485));
#34275=CARTESIAN_POINT('Ctrl Pts',(-0.185685335148621,-0.427093171845309,
-0.187261346324886));
#34276=CARTESIAN_POINT('Ctrl Pts',(0.254072536655689,-0.390300885308689,
-0.175477910677288));
#34277=CARTESIAN_POINT('Ctrl Pts',(0.465701914442558,-0.00306229100798743,
-0.16369447502969));
#34278=CARTESIAN_POINT('Ctrl Pts',(0.259183318990528,0.386925799354961,
-0.151911039382092));
#34279=CARTESIAN_POINT('Ctrl Pts',(-0.180052566671852,0.429498264111241,
-0.140127603734493));
#34280=CARTESIAN_POINT('Ctrl Pts',(-0.457621808803763,0.086429285880465,
-0.128344168086895));
#34281=CARTESIAN_POINT('Ctrl Pts',(-0.3242976250775,-0.33424278860774,-0.116560732439296));
#34282=CARTESIAN_POINT('Ctrl Pts',(0.100208252728578,-0.454803751095683,
-0.104777296791698));
#34283=CARTESIAN_POINT('Ctrl Pts',(0.434740436135497,-0.166999689519078,
-0.0929938611440996));
#34284=CARTESIAN_POINT('Ctrl Pts',(0.378920759912649,0.270746604517297,
-0.0812104254965015));
#34285=CARTESIAN_POINT('Ctrl Pts',(-0.017119674383866,0.465401883275472,
-0.0694269898489029));
#34286=CARTESIAN_POINT('Ctrl Pts',(-0.397802756394656,0.242161554630506,
-0.0576435542013048));
#34287=CARTESIAN_POINT('Ctrl Pts',(-0.42127664327482,-0.1984799085793,-0.0458601185537062));
#34288=CARTESIAN_POINT('Ctrl Pts',(-0.0665433051104071,-0.460971187350655,
-0.0340766829061081));
#34289=CARTESIAN_POINT('Ctrl Pts',(0.348037385925398,-0.309442937396792,
-0.0222932472585096));
#34290=CARTESIAN_POINT('Ctrl Pts',(0.449930166637347,0.119701960714367,
-0.0105098116109113));
#34291=CARTESIAN_POINT('Ctrl Pts',(0.148202710459161,0.441807558502022,
0.00127362403668708));
#34292=CARTESIAN_POINT('Ctrl Pts',(-0.28733267716902,0.366348660462781,
0.0130570596842854));
#34293=CARTESIAN_POINT('Ctrl Pts',(-0.404545717811344,0.0980416532375701,
0.0209126834493509));
#34294=CARTESIAN_POINT('Ctrl Pts',(-0.394131287873257,-0.0316494536977783,
0.0248404953318837));
#34295=CARTESIAN_POINT('',(0.164868911863601,0.359387537208669,-1.11022302462516E-16));
#34296=CARTESIAN_POINT('Ctrl Pts',(0.16490687856217,0.359956139019385,-9.0205620750794E-17));
#34297=CARTESIAN_POINT('Ctrl Pts',(0.15191557524441,0.365209344759306,-8.50453259551574E-17));
#34298=CARTESIAN_POINT('Ctrl Pts',(0.138666480801866,0.36972436752869,-1.12193463301161E-16));
#34299=CARTESIAN_POINT('Ctrl Pts',(0.125198970394113,0.373451590864263,
-7.28583859910259E-17));
#34300=CARTESIAN_POINT('Ctrl Pts',(0.1077614757708,0.378277533811857,-2.52714042912841E-17));
#34301=CARTESIAN_POINT('Ctrl Pts',(0.0899575316801376,0.381783553779889,
-1.1966838214923E-16));
#34302=CARTESIAN_POINT('Ctrl Pts',(0.0719258827732591,0.384004455949837,
-1.2490009027033E-16));
#34303=CARTESIAN_POINT('Ctrl Pts',(0.0653106445601438,0.384819234286422,
-1.26819437505921E-16));
#34304=CARTESIAN_POINT('Ctrl Pts',(0.0586641660849231,0.385460608990607,
-2.41353700608386E-16));
#34305=CARTESIAN_POINT('Ctrl Pts',(0.0520091005880364,0.385929118179874,
-2.22044604925031E-16));
#34306=CARTESIAN_POINT('Ctrl Pts',(0.0301527436928502,0.387467781331137,
-1.58630279885535E-16));
#34307=CARTESIAN_POINT('Ctrl Pts',(0.00816286325548518,0.387151739749051,
-6.77153354539665E-17));
#34308=CARTESIAN_POINT('Ctrl Pts',(-0.0137135983350831,0.385041704764503,
6.93889390390723E-18));
#34309=CARTESIAN_POINT('Ctrl Pts',(-0.0205956652624267,0.384377913596879,
3.04242002786661E-17));
#34310=CARTESIAN_POINT('Ctrl Pts',(-0.0274664476022094,0.383536195767146,
1.30920738496616E-16));
#34311=CARTESIAN_POINT('Ctrl Pts',(-0.0343179685799315,0.382517420028697,
1.2490009027033E-16));
#34312=CARTESIAN_POINT('Ctrl Pts',(-0.0394223585790314,0.381758431081924,
1.20414701304248E-16));
#34313=CARTESIAN_POINT('Ctrl Pts',(-0.0445135904220789,0.380901415994797,
-8.09570049575627E-17));
#34314=CARTESIAN_POINT('Ctrl Pts',(-0.0495799285321691,0.379948761826662,
-7.28583859910259E-17));
#34315=CARTESIAN_POINT('Ctrl Pts',(-0.0708814681958342,0.375943304609374,
-3.88075489983239E-17));
#34316=CARTESIAN_POINT('Ctrl Pts',(-0.0917880441950763,0.370244752838114,
6.22075423807223E-17));
#34317=CARTESIAN_POINT('Ctrl Pts',(-0.112062658453149,0.362907076418133,
3.12250225675825E-17));
#34318=CARTESIAN_POINT('Ctrl Pts',(-0.126357969121762,0.357733396530852,
9.37973661601609E-18));
#34319=CARTESIAN_POINT('Ctrl Pts',(-0.140339041692395,0.351743737927013,
-1.31114297266183E-16));
#34320=CARTESIAN_POINT('Ctrl Pts',(-0.153915171464246,0.344943241496427,
-1.83880688453542E-16));
#34321=CARTESIAN_POINT('Ctrl Pts',(-0.16029905866049,0.341745452227992,
-2.08692965203534E-16));
#34322=CARTESIAN_POINT('Ctrl Pts',(-0.166593284437042,0.33836822022888,
2.86834908564699E-17));
#34323=CARTESIAN_POINT('Ctrl Pts',(-0.172787641053473,0.334811292422105,
3.98986399474666E-17));
#34324=CARTESIAN_POINT('Ctrl Pts',(-0.177212136992572,0.332270655256496,
4.7909380155397E-17));
#34325=CARTESIAN_POINT('Ctrl Pts',(-0.18158449532273,0.329638806505941,
8.55558718079072E-17));
#34326=CARTESIAN_POINT('Ctrl Pts',(-0.185890887386474,0.326922548472184,
9.54097911787244E-17));
#34327=CARTESIAN_POINT('Ctrl Pts',(-0.201503676834758,0.317074777033701,
1.31135095818816E-16));
#34328=CARTESIAN_POINT('Ctrl Pts',(-0.216288937869559,0.306098120574002,
5.49150136144099E-16));
#34329=CARTESIAN_POINT('Ctrl Pts',(-0.230088091924545,0.294011759332474,
3.76434994286967E-16));
#34330=CARTESIAN_POINT('Ctrl Pts',(-0.241247208182782,0.284237746396911,
2.38394309878886E-16));
#34331=CARTESIAN_POINT('Ctrl Pts',(-0.251761185600929,0.273737308875212,
4.47279742850693E-17));
#34332=CARTESIAN_POINT('Ctrl Pts',(-0.261602104460616,0.262589914361208,
1.16226472890446E-16));
#34333=CARTESIAN_POINT('Ctrl Pts',(-0.266706827128519,0.256807491167292,
1.53314473691571E-16));
#34334=CARTESIAN_POINT('Ctrl Pts',(-0.271630267579517,0.250850862471227,
1.68452480644874E-16));
#34335=CARTESIAN_POINT('Ctrl Pts',(-0.276367301437873,0.244730512258966,
2.0122792321331E-16));
#34336=CARTESIAN_POINT('Ctrl Pts',(-0.280626564308997,0.239227452496922,
2.30697677872155E-16));
#34337=CARTESIAN_POINT('Ctrl Pts',(-0.284737477503322,0.233588071488557,
2.55208427141222E-16));
#34338=CARTESIAN_POINT('Ctrl Pts',(-0.288679976022965,0.227844262538324,
2.53269627492614E-16));
#34339=CARTESIAN_POINT('Ctrl Pts',(-0.30046346930519,0.210676942413222,
2.47474867514614E-16));
#34340=CARTESIAN_POINT('Ctrl Pts',(-0.310775801429704,0.192543893686169,
5.6438178067964E-17));
#34341=CARTESIAN_POINT('Ctrl Pts',(-0.319548265568143,0.173669187960367,
9.62771529167128E-17));
#34342=CARTESIAN_POINT('Ctrl Pts',(-0.326817975209212,0.158027786864642,
1.29291568818306E-16));
#34343=CARTESIAN_POINT('Ctrl Pts',(-0.333029562487829,0.141876008150292,
-5.70505344164234E-17));
#34344=CARTESIAN_POINT('Ctrl Pts',(-0.338118323450462,0.125333828641746,
-7.02563007770607E-17));
#34345=CARTESIAN_POINT('Ctrl Pts',(-0.339619932817922,0.120452504505944,
-7.41531044621277E-17));
#34346=CARTESIAN_POINT('Ctrl Pts',(-0.341023607935996,0.115537177016873,
-5.42574854396036E-17));
#34347=CARTESIAN_POINT('Ctrl Pts',(-0.342327260445792,0.110590939653933,
-4.9439619065339E-17));
#34348=CARTESIAN_POINT('Ctrl Pts',(-0.34373737166573,0.105240783266747,
-4.42283166826413E-17));
#34349=CARTESIAN_POINT('Ctrl Pts',(-0.345028225001506,0.0998626025727999,
-1.15077223344712E-16));
#34350=CARTESIAN_POINT('Ctrl Pts',(-0.346197043797798,0.0944662829877048,
-1.06685493772574E-16));
#34351=CARTESIAN_POINT('Ctrl Pts',(-0.350565249921096,0.0742987118212727,
-7.53232290499652E-17));
#34352=CARTESIAN_POINT('Ctrl Pts',(-0.353239911805653,0.0538525131720056,
-1.31602125640592E-16));
#34353=CARTESIAN_POINT('Ctrl Pts',(-0.354123093098514,0.0333368081597991,
-1.83013326715553E-16));
#34354=CARTESIAN_POINT('Ctrl Pts',(-0.355006274391374,0.0128211031475926,
-2.34424527790514E-16));
#34355=CARTESIAN_POINT('Ctrl Pts',(-0.354098424041937,-0.00776559513595167,
-3.76796022219801E-17));
#34356=CARTESIAN_POINT('Ctrl Pts',(-0.351244341336214,-0.0282055544935644,
-1.73472347597681E-18));
#34357=CARTESIAN_POINT('Ctrl Pts',(-0.39480767064478,-0.000104727820695843,
-0.0511159844630761));
#34358=CARTESIAN_POINT('Ctrl Pts',(-0.394952852228362,-0.0583396144091755,
-0.0493640291599528));
#34359=CARTESIAN_POINT('Ctrl Pts',(-0.382867850318616,-0.116517499431679,
-0.0476120738568295));
#34360=CARTESIAN_POINT('Ctrl Pts',(-0.35824210576739,-0.168788211172892,
-0.0458601185537063));
#34361=CARTESIAN_POINT('Ctrl Pts',(-0.303032197220016,-0.285977001503084,
-0.0419323066711736));
#34362=CARTESIAN_POINT('Ctrl Pts',(-0.18478775116521,-0.37347409442687,
-0.0380044947886408));
#34363=CARTESIAN_POINT('Ctrl Pts',(-0.0565687462985088,-0.391967932563119,
-0.034076682906108));
#34364=CARTESIAN_POINT('Ctrl Pts',(0.0716502585681938,-0.410461770699368,
-0.0301488710235753));
#34365=CARTESIAN_POINT('Ctrl Pts',(0.209843822246795,-0.35995235404808,
-0.0262210591410425));
#34366=CARTESIAN_POINT('Ctrl Pts',(0.295922734204754,-0.263173496037244,
-0.0222932472585097));
#34367=CARTESIAN_POINT('Ctrl Pts',(0.382001646162714,-0.166394638026406,
-0.0183654353759768));
#34368=CARTESIAN_POINT('Ctrl Pts',(0.415965906400031,-0.023346338656019,
-0.0144376234934441));
#34369=CARTESIAN_POINT('Ctrl Pts',(0.382660127155657,0.101862077327118,
-0.0105098116109112));
#34370=CARTESIAN_POINT('Ctrl Pts',(0.35295423526798,0.213537220590751,-0.00700654107394087));
#34371=CARTESIAN_POINT('Ctrl Pts',(0.26973431106858,0.31102054676347,-0.00350327053697048));
#34372=CARTESIAN_POINT('Ctrl Pts',(0.16490687856217,0.359956139019385,-9.0205620750794E-17));
#34373=CARTESIAN_POINT('',(0.200169762396267,-0.290577011776231,-0.8));
#34374=CARTESIAN_POINT('Ctrl Pts',(0.20016976239627,-0.290577011776229,
-0.8));
#34375=CARTESIAN_POINT('Ctrl Pts',(0.190306482557462,-0.298378649280142,
-0.8));
#34376=CARTESIAN_POINT('Ctrl Pts',(0.180035217986072,-0.305605974903153,
-0.8));
#34377=CARTESIAN_POINT('Ctrl Pts',(0.169385277865962,-0.312209719032721,
-0.8));
#34378=CARTESIAN_POINT('Ctrl Pts',(0.15368545462129,-0.321944761147323,
-0.8));
#34379=CARTESIAN_POINT('Ctrl Pts',(0.137163515983412,-0.330326466268722,
-0.8));
#34380=CARTESIAN_POINT('Ctrl Pts',(0.120002461186164,-0.337372376845852,
-0.8));
#34381=CARTESIAN_POINT('Ctrl Pts',(0.114202478233197,-0.339753708396756,
-0.8));
#34382=CARTESIAN_POINT('Ctrl Pts',(0.108338590630642,-0.341978348949641,
-0.8));
#34383=CARTESIAN_POINT('Ctrl Pts',(0.102419584724057,-0.344047141145212,
-0.8));
#34384=CARTESIAN_POINT('Ctrl Pts',(0.0863681048207357,-0.349657403556746,
-0.8));
#34385=CARTESIAN_POINT('Ctrl Pts',(0.0699088827807137,-0.354124467710462,
-0.8));
#34386=CARTESIAN_POINT('Ctrl Pts',(0.0531808102711496,-0.357460993149358,
-0.8));
#34387=CARTESIAN_POINT('Ctrl Pts',(0.0464251329711486,-0.358808457966691,
-0.8));
#34388=CARTESIAN_POINT('Ctrl Pts',(0.0396254752335136,-0.359971281620787,
-0.8));
#34389=CARTESIAN_POINT('Ctrl Pts',(0.0327905864186719,-0.360949250929142,
-0.8));
#34390=CARTESIAN_POINT('Ctrl Pts',(0.0272161405436249,-0.361746869899189,
-0.8));
#34391=CARTESIAN_POINT('Ctrl Pts',(0.021618656359546,-0.362421254066241,
-0.8));
#34392=CARTESIAN_POINT('Ctrl Pts',(0.0160166140773693,-0.362971297712489,
-0.8));
#34393=CARTESIAN_POINT('Ctrl Pts',(-0.00503455293683043,-0.36503823331901,
-0.8));
#34394=CARTESIAN_POINT('Ctrl Pts',(-0.0261975225172284,-0.365360927269529,
-0.8));
#34395=CARTESIAN_POINT('Ctrl Pts',(-0.0472196904885675,-0.363958480743644,
-0.8));
#34396=CARTESIAN_POINT('Ctrl Pts',(-0.0621644164904353,-0.362961477052578,
-0.8));
#34397=CARTESIAN_POINT('Ctrl Pts',(-0.0770386390163482,-0.361091594946764,
-0.8));
#34398=CARTESIAN_POINT('Ctrl Pts',(-0.0917535281674465,-0.358339847735959,
-0.8));
#34399=CARTESIAN_POINT('Ctrl Pts',(-0.098600486653832,-0.357059437212716,
-0.8));
#34400=CARTESIAN_POINT('Ctrl Pts',(-0.105412934492697,-0.355587902723317,
-0.8));
#34401=CARTESIAN_POINT('Ctrl Pts',(-0.112181716986231,-0.353923330911631,
-0.8));
#34402=CARTESIAN_POINT('Ctrl Pts',(-0.116968091051461,-0.352746270878047,
-0.8));
#34403=CARTESIAN_POINT('Ctrl Pts',(-0.12172870669558,-0.351473523653454,
-0.8));
#34404=CARTESIAN_POINT('Ctrl Pts',(-0.126452665500413,-0.350107261479429,
-0.8));
#34405=CARTESIAN_POINT('Ctrl Pts',(-0.143772909154477,-0.345097904978429,
-0.8));
#34406=CARTESIAN_POINT('Ctrl Pts',(-0.160631985153867,-0.338825890448156,
-0.8));
#34407=CARTESIAN_POINT('Ctrl Pts',(-0.176878423079808,-0.331288354642354,
-0.8));
#34408=CARTESIAN_POINT('Ctrl Pts',(-0.191156219349634,-0.324664170245606,
-0.8));
#34409=CARTESIAN_POINT('Ctrl Pts',(-0.204961220157989,-0.317062223203108,
-0.8));
#34410=CARTESIAN_POINT('Ctrl Pts',(-0.218247963486141,-0.308569468881161,
-0.8));
#34411=CARTESIAN_POINT('Ctrl Pts',(-0.224802936957718,-0.304379594966531,
-0.8));
#34412=CARTESIAN_POINT('Ctrl Pts',(-0.231231666263234,-0.299972654194668,
-0.8));
#34413=CARTESIAN_POINT('Ctrl Pts',(-0.237527947545455,-0.295357764267163,
-0.8));
#34414=CARTESIAN_POINT('Ctrl Pts',(-0.242759499159343,-0.291523273118186,
-0.8));
#34415=CARTESIAN_POINT('Ctrl Pts',(-0.247901647723441,-0.287543179968104,
-0.8));
#34416=CARTESIAN_POINT('Ctrl Pts',(-0.252932096788435,-0.283438407946873,
-0.8));
#34417=CARTESIAN_POINT('Ctrl Pts',(-0.269421005257647,-0.269983702557636,
-0.8));
#34418=CARTESIAN_POINT('Ctrl Pts',(-0.284755423501557,-0.255163052021068,
-0.8));
#34419=CARTESIAN_POINT('Ctrl Pts',(-0.298831470631119,-0.239191762115533,
-0.8));
#34420=CARTESIAN_POINT('Ctrl Pts',(-0.311279850930076,-0.225067293166332,
-0.8));
#34421=CARTESIAN_POINT('Ctrl Pts',(-0.322744216465833,-0.210041634577153,
-0.8));
#34422=CARTESIAN_POINT('Ctrl Pts',(-0.333132984278499,-0.194238114040248,
-0.8));
#34423=CARTESIAN_POINT('Ctrl Pts',(-0.336326088260912,-0.189380725245687,
-0.8));
#34424=CARTESIAN_POINT('Ctrl Pts',(-0.339417416663507,-0.184449716680632,
-0.8));
#34425=CARTESIAN_POINT('Ctrl Pts',(-0.342403840382252,-0.179448352887251,
-0.8));
#34426=CARTESIAN_POINT('Ctrl Pts',(-0.345031246832228,-0.175048235312868,
-0.8));
#34427=CARTESIAN_POINT('Ctrl Pts',(-0.347572530726044,-0.170601882868889,
-0.8));
#34428=CARTESIAN_POINT('Ctrl Pts',(-0.350026053733772,-0.166112593145433,
-0.8));
#34429=CARTESIAN_POINT('Ctrl Pts',(-0.361014852315233,-0.146006036007191,
-0.8));
#34430=CARTESIAN_POINT('Ctrl Pts',(-0.370248738553699,-0.125038049791925,
-0.8));
#34431=CARTESIAN_POINT('Ctrl Pts',(-0.377580893333559,-0.103434617138351,
-0.8));
#34432=CARTESIAN_POINT('Ctrl Pts',(-0.384469721870555,-0.0831373992223077,
-0.8));
#34433=CARTESIAN_POINT('Ctrl Pts',(-0.38968034295518,-0.062277824821227,
-0.8));
#34434=CARTESIAN_POINT('Ctrl Pts',(-0.393046362175399,-0.0410217592765385,
-0.8));
#34435=CARTESIAN_POINT('Ctrl Pts',(-0.393262980232635,-0.0396538385008335,
-0.8));
#34436=CARTESIAN_POINT('Ctrl Pts',(-0.393471941134707,-0.0382842719653916,
-0.8));
#34437=CARTESIAN_POINT('Ctrl Pts',(-0.393673192958032,-0.0369131026361633,
-0.8));
#34438=CARTESIAN_POINT('Ctrl Pts',(0.200169762396267,-0.290577011776231,
-0.8));
#34439=CARTESIAN_POINT('Ctrl Pts',(0.284652167513286,-0.231483393422286,
-0.79649672946303));
#34440=CARTESIAN_POINT('Ctrl Pts',(0.407768891830231,-0.0227977591064635,
-0.789065647043525));
#34441=CARTESIAN_POINT('Ctrl Pts',(0.257863027527083,0.32520678286678,-0.777706752741491));
#34442=CARTESIAN_POINT('Ctrl Pts',(-0.129379073725142,0.394390194728457,
-0.765923317093891));
#34443=CARTESIAN_POINT('Ctrl Pts',(-0.334426670897645,0.178706874259964,
-0.757006559445049));
#34444=CARTESIAN_POINT('Ctrl Pts',(-0.352510997026901,0.0316401701347851,
-0.752017613678738));
#34445=CARTESIAN_POINT('Ctrl Pts',(-0.352246168648579,0.000295985828685053,
-0.75095647979496));
#34446=CARTESIAN_POINT('Origin',(-9.39637619619865E-17,-2.12715743287418E-17,
-0.8));
#34447=CARTESIAN_POINT('',(0.339445800272064,0.0945763675695885,-0.8));
#34448=CARTESIAN_POINT('Ctrl Pts',(-0.278859905177389,0.281069071148119,
-0.800000000000001));
#34449=CARTESIAN_POINT('Ctrl Pts',(-0.268475009873748,0.290477793453348,
-0.800000000000001));
#34450=CARTESIAN_POINT('Ctrl Pts',(-0.25759371033593,0.29928240376613,-0.800000000000001));
#34451=CARTESIAN_POINT('Ctrl Pts',(-0.24623586993354,0.307422754976269,
-0.800000000000001));
#34452=CARTESIAN_POINT('Ctrl Pts',(-0.231529933077798,0.317962742037073,
-0.800000000000001));
#34453=CARTESIAN_POINT('Ctrl Pts',(-0.216025100159335,0.327389965026806,
-0.8));
#34454=CARTESIAN_POINT('Ctrl Pts',(-0.199863609434863,0.335689279670645,
-0.8));
#34455=CARTESIAN_POINT('Ctrl Pts',(-0.193934478213887,0.33873403132174,
-0.8));
#34456=CARTESIAN_POINT('Ctrl Pts',(-0.187916258974387,0.341626769901992,
-0.8));
#34457=CARTESIAN_POINT('Ctrl Pts',(-0.181830402402309,0.344360193317562,
-0.8));
#34458=CARTESIAN_POINT('Ctrl Pts',(-0.161843412934983,0.353337221344707,
-0.8));
#34459=CARTESIAN_POINT('Ctrl Pts',(-0.1410918738637,0.360619192332112,-0.8));
#34460=CARTESIAN_POINT('Ctrl Pts',(-0.119828519294813,0.366177991655667,
-0.8));
#34461=CARTESIAN_POINT('Ctrl Pts',(-0.113139294026385,0.367926730819884,
-0.8));
#34462=CARTESIAN_POINT('Ctrl Pts',(-0.106399340447922,0.369504553265394,
-0.8));
#34463=CARTESIAN_POINT('Ctrl Pts',(-0.0996164460696241,0.370909525367399,
-0.8));
#34464=CARTESIAN_POINT('Ctrl Pts',(-0.094563178597882,0.371956231894996,
-0.8));
#34465=CARTESIAN_POINT('Ctrl Pts',(-0.0894884791182313,0.372906381891583,
-0.8));
#34466=CARTESIAN_POINT('Ctrl Pts',(-0.0844041867529184,0.37375817163292,
-0.8));
#34467=CARTESIAN_POINT('Ctrl Pts',(-0.0630272839706001,0.377339520851892,
-0.8));
#34468=CARTESIAN_POINT('Ctrl Pts',(-0.0414376343613116,0.379195383149306,
-0.8));
#34469=CARTESIAN_POINT('Ctrl Pts',(-0.0198763137447139,0.37929474254576,
-0.8));
#34470=CARTESIAN_POINT('Ctrl Pts',(-0.00467371801110023,0.37936479951321,
-0.8));
#34471=CARTESIAN_POINT('Ctrl Pts',(0.0105151140659063,0.378560564121899,
-0.8));
#34472=CARTESIAN_POINT('Ctrl Pts',(0.0256032632385705,0.376855601414503,
-0.8));
#34473=CARTESIAN_POINT('Ctrl Pts',(0.0326988428047688,0.376053800053098,
-0.8));
#34474=CARTESIAN_POINT('Ctrl Pts',(0.039772093686793,0.375052608106074,
-0.8));
#34475=CARTESIAN_POINT('Ctrl Pts',(0.0468135179423963,0.373848268808225,
-0.8));
#34476=CARTESIAN_POINT('Ctrl Pts',(0.0518424079668323,0.372988145960754,
-0.8));
#34477=CARTESIAN_POINT('Ctrl Pts',(0.0568537870825205,0.372024437031212,
-0.8));
#34478=CARTESIAN_POINT('Ctrl Pts',(0.0618323347754462,0.370958760988685,
-0.8));
#34479=CARTESIAN_POINT('Ctrl Pts',(0.0798818210244701,0.36709520352938,
-0.8));
#34480=CARTESIAN_POINT('Ctrl Pts',(0.0975435693854742,0.361886824549212,
-0.8));
#34481=CARTESIAN_POINT('Ctrl Pts',(0.114662125904877,0.355296980178815,
-0.8));
#34482=CARTESIAN_POINT('Ctrl Pts',(0.128506110242191,0.34996769308935,-0.8));
#34483=CARTESIAN_POINT('Ctrl Pts',(0.141994842420674,0.343734144970146,
-0.8));
#34484=CARTESIAN_POINT('Ctrl Pts',(0.155074724264531,0.33666131221326,-0.8));
#34485=CARTESIAN_POINT('Ctrl Pts',(0.161859575051541,0.332992462947662,
-0.8));
#34486=CARTESIAN_POINT('Ctrl Pts',(0.168534289696369,0.329097603646923,
-0.8));
#34487=CARTESIAN_POINT('Ctrl Pts',(0.175090444399602,0.324984809875769,
-0.8));
#34488=CARTESIAN_POINT('Ctrl Pts',(0.180985353825959,0.321286827160645,
-0.8));
#34489=CARTESIAN_POINT('Ctrl Pts',(0.186787985179493,0.317409747559543,
-0.8));
#34490=CARTESIAN_POINT('Ctrl Pts',(0.192468510837425,0.313376595109622,
-0.8));
#34491=CARTESIAN_POINT('Ctrl Pts',(0.2094466944668,0.301322146802642,-0.8));
#34492=CARTESIAN_POINT('Ctrl Pts',(0.225376684523978,0.287854111002053,
-0.8));
#34493=CARTESIAN_POINT('Ctrl Pts',(0.240116755803838,0.273159151623289,
-0.8));
#34494=CARTESIAN_POINT('Ctrl Pts',(0.252331794876079,0.260981496605985,
-0.8));
#34495=CARTESIAN_POINT('Ctrl Pts',(0.263729437817635,0.247960058877349,
-0.8));
#34496=CARTESIAN_POINT('Ctrl Pts',(0.274207594017334,0.234185164645355,
-0.8));
#34497=CARTESIAN_POINT('Ctrl Pts',(0.277299531732945,0.230120411821221,
-0.8));
#34498=CARTESIAN_POINT('Ctrl Pts',(0.280311253869966,0.225989986271888,
-0.8));
#34499=CARTESIAN_POINT('Ctrl Pts',(0.283239733805565,0.221796072218523,
-0.8));
#34500=CARTESIAN_POINT('Ctrl Pts',(0.286407344655221,0.217259695685267,
-0.8));
#34501=CARTESIAN_POINT('Ctrl Pts',(0.289472662759133,0.212655910806126,
-0.8));
#34502=CARTESIAN_POINT('Ctrl Pts',(0.292429674704035,0.207993040211104,
-0.8));
#34503=CARTESIAN_POINT('Ctrl Pts',(0.303480889882578,0.190566534246487,
-0.8));
#34504=CARTESIAN_POINT('Ctrl Pts',(0.313038342233419,0.172294802880286,
-0.8));
#34505=CARTESIAN_POINT('Ctrl Pts',(0.320938020590327,0.153340401549331,
-0.8));
#34506=CARTESIAN_POINT('Ctrl Pts',(0.328837698947234,0.134386000218375,
-0.8));
#34507=CARTESIAN_POINT('Ctrl Pts',(0.335080537221356,0.114747687841751,
-0.8));
#34508=CARTESIAN_POINT('Ctrl Pts',(0.339445800272064,0.0945763675695893,
-0.8));
#34509=CARTESIAN_POINT('Origin',(0.,0.,-0.8));
#34510=CARTESIAN_POINT('Origin',(0.,0.,-0.953243520205039));
#34511=CARTESIAN_POINT('Ctrl Pts',(0.339445800272064,0.094576367569588,
-0.8));
#34512=CARTESIAN_POINT('Ctrl Pts',(0.308324917009509,0.206272908636879,
-0.796072188117467));
#34513=CARTESIAN_POINT('Ctrl Pts',(0.12785742430771,0.394733928544834,-0.788216564352402));
#34514=CARTESIAN_POINT('Ctrl Pts',(-0.247689876721063,0.326277103430375,
-0.776797737754082));
#34515=CARTESIAN_POINT('Ctrl Pts',(-0.352173024012217,0.104655642871124,
-0.769306723038295));
#34516=CARTESIAN_POINT('Ctrl Pts',(-0.352786263833399,-0.000190149253296124,
-0.76574352020504));
#34517=CARTESIAN_POINT('Ctrl Pts',(0.380892144526639,0.106124145404794,
-0.824840495331884));
#34518=CARTESIAN_POINT('Ctrl Pts',(0.345971400313757,0.231458838098676,
-0.820912683449351));
#34519=CARTESIAN_POINT('Ctrl Pts',(0.143468820351243,0.44293095522278,-0.813057059684284));
#34520=CARTESIAN_POINT('Ctrl Pts',(-0.291388392138657,0.363662793626005,
-0.801273624036688));
#34521=CARTESIAN_POINT('Ctrl Pts',(-0.46361938361485,-0.042696984818944,
-0.789490188389088));
#34522=CARTESIAN_POINT('Ctrl Pts',(-0.220067036752125,-0.410433220025444,
-0.77770675274149));
#34523=CARTESIAN_POINT('Ctrl Pts',(0.221336844762247,-0.409795607414138,
-0.765923317093893));
#34524=CARTESIAN_POINT('Ctrl Pts',(0.463871431563072,-0.0411298069848769,
-0.754139881446293));
#34525=CARTESIAN_POINT('Ctrl Pts',(0.289971644477912,0.364425190131086,
-0.742356445798696));
#34526=CARTESIAN_POINT('Ctrl Pts',(-0.144326642460796,0.442788711872689,
-0.730573010151097));
#34527=CARTESIAN_POINT('Ctrl Pts',(-0.449016693789206,0.123566658604731,
-0.7187895745035));
#34528=CARTESIAN_POINT('Ctrl Pts',(-0.350550328424412,-0.30659850382061,
-0.7070061388559));
#34529=CARTESIAN_POINT('Ctrl Pts',(0.0626760165915523,-0.461475781257629,
-0.695222703208302));
#34530=CARTESIAN_POINT('Ctrl Pts',(0.419623607977338,-0.201998157742978,
-0.683439267560704));
#34531=CARTESIAN_POINT('Ctrl Pts',(0.39979787554505,0.238850234477996,-0.671655831913105));
#34532=CARTESIAN_POINT('Ctrl Pts',(0.0209979054846499,0.465238442645313,
-0.659872396265508));
#34533=CARTESIAN_POINT('Ctrl Pts',(-0.376655426161442,0.273894673808823,
-0.648088960617908));
#34534=CARTESIAN_POINT('Ctrl Pts',(-0.436114792825645,-0.163375558641342,
-0.636305524970311));
#34535=CARTESIAN_POINT('Ctrl Pts',(-0.103992062925303,-0.453952994102977,
-0.624522089322712));
#34536=CARTESIAN_POINT('Ctrl Pts',(0.321503776225126,-0.336931711343498,
-0.612738653675114));
#34537=CARTESIAN_POINT('Ctrl Pts',(0.458325446868897,0.082616301207692,
-0.600955218027515));
#34538=CARTESIAN_POINT('Ctrl Pts',(0.183622446346355,0.427984184736038,
-0.589171782379917));
#34539=CARTESIAN_POINT('Ctrl Pts',(-0.255952831769196,0.38907044560016,
-0.577388346732319));
#34540=CARTESIAN_POINT('Ctrl Pts',(-0.465711284854635,0.000815248043422982,
-0.565604911084721));
#34541=CARTESIAN_POINT('Ctrl Pts',(-0.257313428960664,-0.388171951771344,
-0.553821475437122));
#34542=CARTESIAN_POINT('Ctrl Pts',(0.182122918148132,-0.428624436334322,
-0.542038039789524));
#34543=CARTESIAN_POINT('Ctrl Pts',(0.45803338769357,-0.0842204294398452,
-0.530254604141926));
#34544=CARTESIAN_POINT('Ctrl Pts',(0.322681437476349,0.335804042236243,
-0.518471168494327));
#34545=CARTESIAN_POINT('Ctrl Pts',(-0.10240211785065,0.454314286730666,
-0.506687732846729));
#34546=CARTESIAN_POINT('Ctrl Pts',(-0.435540099262727,0.164901445821025,
-0.49490429719913));
#34547=CARTESIAN_POINT('Ctrl Pts',(-0.377612102033148,-0.272574329827866,
-0.483120861551532));
#34548=CARTESIAN_POINT('Ctrl Pts',(0.0193690534496328,-0.465309042091788,
-0.471337425903934));
#34549=CARTESIAN_POINT('Ctrl Pts',(0.398958979401207,-0.24024861631879,
-0.459553990256335));
#34550=CARTESIAN_POINT('Ctrl Pts',(0.420328654298526,0.200528021136553,
-0.447770554608737));
#34551=CARTESIAN_POINT('Ctrl Pts',(0.064290515766074,0.461253069874142,
-0.435987118961139));
#34552=CARTESIAN_POINT('Ctrl Pts',(-0.349473268478174,0.307824787022427,
-0.42420368331354));
#34553=CARTESIAN_POINT('Ctrl Pts',(-0.449449399272338,-0.121995501472316,
-0.412420247665942));
#34554=CARTESIAN_POINT('Ctrl Pts',(-0.145870565889691,-0.442277563180907,
-0.400636812018343));
#34555=CARTESIAN_POINT('Ctrl Pts',(0.288683614412624,-0.36544416215812,
-0.388853376370746));
#34556=CARTESIAN_POINT('Ctrl Pts',(0.46403240727406,0.0395169569272912,
-0.377069940723147));
#34557=CARTESIAN_POINT('Ctrl Pts',(0.222732336443623,0.408996297281908,
-0.365286505075549));
#34558=CARTESIAN_POINT('Ctrl Pts',(-0.218556298620971,0.41124300506758,
-0.35350306942795));
#34559=CARTESIAN_POINT('Ctrl Pts',(-0.463605981299019,0.0442397896330434,
-0.341719633780352));
#34560=CARTESIAN_POINT('Ctrl Pts',(-0.292389682817799,-0.362485776660763,
-0.329936198132754));
#34561=CARTESIAN_POINT('Ctrl Pts',(0.14135963534951,-0.443739921983301,
-0.318152762485155));
#34562=CARTESIAN_POINT('Ctrl Pts',(0.448183914359544,-0.126565571082187,
-0.306369326837557));
#34563=CARTESIAN_POINT('Ctrl Pts',(0.352589492277338,0.304250414811037,
-0.294585891189958));
#34564=CARTESIAN_POINT('Ctrl Pts',(-0.0595906015999328,0.461883778605252,
-0.28280245554236));
#34565=CARTESIAN_POINT('Ctrl Pts',(-0.418265043254798,0.204797505982204,
-0.271019019894762));
#34566=CARTESIAN_POINT('Ctrl Pts',(-0.40138456254368,-0.236173873283955,
-0.259235584247163));
#34567=CARTESIAN_POINT('Ctrl Pts',(-0.024105928921317,-0.465087699171906,
-0.247452148599566));
#34568=CARTESIAN_POINT('Ctrl Pts',(0.374817112762246,-0.276405132309377,
-0.235668712951966));
#34569=CARTESIAN_POINT('Ctrl Pts',(0.437196586488692,0.160458135460469,
-0.223885277304369));
#34570=CARTESIAN_POINT('Ctrl Pts',(0.107022733782069,0.45324804543394,-0.21210184165677));
#34571=CARTESIAN_POINT('Ctrl Pts',(-0.319245469084403,0.339072264385629,
-0.200318406009172));
#34572=CARTESIAN_POINT('Ctrl Pts',(-0.458867211564245,-0.0795522962206605,
-0.188534970361574));
#34573=CARTESIAN_POINT('Ctrl Pts',(-0.186477793345172,-0.426747741630595,
-0.176751534713975));
#34574=CARTESIAN_POINT('Ctrl Pts',(0.253347573627205,-0.390771963537543,
-0.164968099066377));
#34575=CARTESIAN_POINT('Ctrl Pts',(0.465695563601222,-0.00392655608262027,
-0.153184663418778));
#34576=CARTESIAN_POINT('Ctrl Pts',(0.259900935227136,0.386443698320385,
-0.14140122777118));
#34577=CARTESIAN_POINT('Ctrl Pts',(-0.179254658034234,0.429832464241771,
-0.129617792123582));
#34578=CARTESIAN_POINT('Ctrl Pts',(-0.457461308535371,0.087277296570209,
-0.117834356475983));
#34579=CARTESIAN_POINT('Ctrl Pts',(-0.324916220195966,-0.333637768056457,
-0.106050920828385));
#34580=CARTESIAN_POINT('Ctrl Pts',(0.0993613588387723,-0.454993783974677,
-0.0942674851807868));
#34581=CARTESIAN_POINT('Ctrl Pts',(0.434434510205315,-0.167797288851672,
-0.0824840495331884));
#34582=CARTESIAN_POINT('Ctrl Pts',(0.379413574932619,0.270025378806949,
-0.07070061388559));
#34583=CARTESIAN_POINT('Ctrl Pts',(-0.0162382856254888,0.4654661714724,
-0.0589171782379918));
#34584=CARTESIAN_POINT('Ctrl Pts',(-0.397385996561566,0.242835949772861,
-0.0471337425903934));
#34585=CARTESIAN_POINT('Ctrl Pts',(-0.421580183389628,-0.197575591481363,
-0.035350306942795));
#34586=CARTESIAN_POINT('Ctrl Pts',(-0.0675247742952343,-0.461083753126696,
-0.0235668712951966));
#34587=CARTESIAN_POINT('Ctrl Pts',(0.347731504741513,-0.309602865163979,
-0.0117834356475983));
#34588=CARTESIAN_POINT('Ctrl Pts',(0.41551906970067,-0.0247650213838164,
-0.00392781188253288));
#34589=CARTESIAN_POINT('Ctrl Pts',(0.382276194676387,0.101025100760854,
-1.11022302462516E-16));
#34590=CARTESIAN_POINT('Ctrl Pts',(0.367076696441781,0.102274886126392,
-0.816560330221256));
#34591=CARTESIAN_POINT('Ctrl Pts',(0.333422572545675,0.223063528278077,
-0.812632518338723));
#34592=CARTESIAN_POINT('Ctrl Pts',(0.138265021670065,0.426865279663465,
-0.804776894573656));
#34593=CARTESIAN_POINT('Ctrl Pts',(-0.280819360295995,0.3504722762632,-0.792993458926061));
#34594=CARTESIAN_POINT('Ctrl Pts',(-0.446803312142898,-0.0411483102515571,
-0.78121002327846));
#34595=CARTESIAN_POINT('Ctrl Pts',(-0.212084922221472,-0.395546279128804,
-0.769426587630863));
#34596=CARTESIAN_POINT('Ctrl Pts',(0.21330867266151,-0.394931793547173,
-0.757643151983265));
#34597=CARTESIAN_POINT('Ctrl Pts',(0.447046217987789,-0.0396379759736438,
-0.745859716335665));
#34598=CARTESIAN_POINT('Ctrl Pts',(0.279453999895495,0.351207019666249,
-0.734076280688068));
#34599=CARTESIAN_POINT('Ctrl Pts',(-0.139091729468151,0.426728195662672,
-0.72229284504047));
#34600=CARTESIAN_POINT('Ctrl Pts',(-0.432730280663021,0.119084736933454,
-0.710509409392871));
#34601=CARTESIAN_POINT('Ctrl Pts',(-0.337835417043143,-0.295477781660029,
-0.698725973745272));
#34602=CARTESIAN_POINT('Ctrl Pts',(0.0604026768395285,-0.444737461000834,
-0.686942538097675));
#34603=CARTESIAN_POINT('Ctrl Pts',(0.404403319886607,-0.194671424698894,
-0.675159102450075));
#34604=CARTESIAN_POINT('Ctrl Pts',(0.385296692274669,0.230186829201976,
-0.663375666802478));
#34605=CARTESIAN_POINT('Ctrl Pts',(0.0202362844397346,0.44836364581947,
-0.651592231154879));
#34606=CARTESIAN_POINT('Ctrl Pts',(-0.362993649302062,0.26396016163497,
-0.639808795507281));
#34607=CARTESIAN_POINT('Ctrl Pts',(-0.420296348245201,-0.157449716953142,
-0.628025359859683));
#34608=CARTESIAN_POINT('Ctrl Pts',(-0.100220137021271,-0.437487535014054,
-0.616241924212084));
#34609=CARTESIAN_POINT('Ctrl Pts',(0.309842420659382,-0.324710764723573,
-0.604458488564485));
#34610=CARTESIAN_POINT('Ctrl Pts',(0.441701393293164,0.0796197016802426,
-0.592675052916888));
#34611=CARTESIAN_POINT('Ctrl Pts',(0.176962223994262,0.412460647770714,
-0.580891617269289));
#34612=CARTESIAN_POINT('Ctrl Pts',(-0.2466690932876,0.3749583600143,-0.569108181621692));
#34613=CARTESIAN_POINT('Ctrl Pts',(-0.448819337433567,0.000785677948102577,
-0.557324745974092));
#34614=CARTESIAN_POINT('Ctrl Pts',(-0.247980339868577,-0.374092455712532,
-0.545541310326495));
#34615=CARTESIAN_POINT('Ctrl Pts',(0.175517085612874,-0.413077676619869,
-0.533757874678895));
#34616=CARTESIAN_POINT('Ctrl Pts',(0.441419927479849,-0.0811656461177657,
-0.521974439031298));
#34617=CARTESIAN_POINT('Ctrl Pts',(0.310977366622007,0.323623997625541,
-0.510191003383699));
#34618=CARTESIAN_POINT('Ctrl Pts',(-0.0986878612998801,0.437835723093348,
-0.498407567736101));
#34619=CARTESIAN_POINT('Ctrl Pts',(-0.419742499557131,0.158920258241822,
-0.486624132088502));
#34620=CARTESIAN_POINT('Ctrl Pts',(-0.363915625309175,-0.262687708228774,
-0.474840696440904));
#34621=CARTESIAN_POINT('Ctrl Pts',(0.0186665129634842,-0.448431684533198,
-0.463057260793306));
#34622=CARTESIAN_POINT('Ctrl Pts',(0.384488223973171,-0.231534489934439,
-0.451273825145707));
#34623=CARTESIAN_POINT('Ctrl Pts',(0.405082793270711,0.193254611838459,
-0.439490389498109));
#34624=CARTESIAN_POINT('Ctrl Pts',(0.0619586160519983,0.444522827645736,
-0.427706953850511));
#34625=CARTESIAN_POINT('Ctrl Pts',(-0.336797423446752,0.296659585992549,
-0.415923518202913));
#34626=CARTESIAN_POINT('Ctrl Pts',(-0.43314729136162,-0.117570567691465,
-0.404140082555314));
#34627=CARTESIAN_POINT('Ctrl Pts',(-0.140579652808082,-0.426235586991514,
-0.392356646907716));
#34628=CARTESIAN_POINT('Ctrl Pts',(0.278212688337677,-0.352189032266994,
-0.380573211260117));
#34629=CARTESIAN_POINT('Ctrl Pts',(0.44720135490265,0.0380836260625165,
-0.36878977561252));
#34630=CARTESIAN_POINT('Ctrl Pts',(0.214653548064355,0.394161475421722,
-0.35700633996492));
#34631=CARTESIAN_POINT('Ctrl Pts',(-0.210628980505842,0.396326692225704,
-0.345222904317323));
#34632=CARTESIAN_POINT('Ctrl Pts',(-0.446790395946305,0.0426351555502902,
-0.333439468669723));
#34633=CARTESIAN_POINT('Ctrl Pts',(-0.281784332874083,-0.349337951217475,
-0.321656033022126));
#34634=CARTESIAN_POINT('Ctrl Pts',(0.136232339521731,-0.427644904158876,
-0.309872597374527));
#34635=CARTESIAN_POINT('Ctrl Pts',(0.431927707214611,-0.121974874997368,
-0.298089161726929));
#34636=CARTESIAN_POINT('Ctrl Pts',(0.339800617799819,0.293214860859558,
-0.28630572607933));
#34637=CARTESIAN_POINT('Ctrl Pts',(-0.0574291738189212,0.445130659759787,
-0.274522290431733));
#34638=CARTESIAN_POINT('Ctrl Pts',(-0.403094032054294,0.197369236976231,
-0.262738854784134));
#34639=CARTESIAN_POINT('Ctrl Pts',(-0.386825828094648,-0.227607543071477,
-0.250955419136536));
#34640=CARTESIAN_POINT('Ctrl Pts',(-0.0232315758680031,-0.44821837000577,
-0.239171983488938));
#34641=CARTESIAN_POINT('Ctrl Pts',(0.361222013894774,-0.266379562576102,
-0.227388547841339));
#34642=CARTESIAN_POINT('Ctrl Pts',(0.421338903860403,0.154638112464191,
-0.215605112193741));
#34643=CARTESIAN_POINT('Ctrl Pts',(0.103140881547223,0.436808155740133,
-0.203821676546142));
#34644=CARTESIAN_POINT('Ctrl Pts',(-0.307666025223877,0.326773677153128,
-0.192038240898544));
#34645=CARTESIAN_POINT('Ctrl Pts',(-0.442223507486053,-0.0766668320958137,
-0.180254805250946));
#34646=CARTESIAN_POINT('Ctrl Pts',(-0.179714003884139,-0.411269052047342,
-0.168471369603347));
#34647=CARTESIAN_POINT('Ctrl Pts',(0.244158331209982,-0.376598161707157,
-0.156687933955749));
#34648=CARTESIAN_POINT('Ctrl Pts',(0.44880418641024,-0.00378413484214192,
-0.144904498308151));
#34649=CARTESIAN_POINT('Ctrl Pts',(0.250473993954038,0.372426888237571,
-0.133121062660552));
#34650=CARTESIAN_POINT('Ctrl Pts',(-0.172752860983212,0.414241887801034,
-0.121337627012954));
#34651=CARTESIAN_POINT('Ctrl Pts',(-0.440868598368676,0.0841116367447717,
-0.109554191365355));
#34652=CARTESIAN_POINT('Ctrl Pts',(-0.313131090897422,-0.321536296997084,
-0.0977707557177573));
#34653=CARTESIAN_POINT('Ctrl Pts',(0.0957573945291805,-0.438490574098172,
-0.0859873200701589));
#34654=CARTESIAN_POINT('Ctrl Pts',(0.418677011637128,-0.161711065320358,
-0.0742038844225605));
#34655=CARTESIAN_POINT('Ctrl Pts',(0.365651756469058,0.260231210940511,
-0.062420448774962));
#34656=CARTESIAN_POINT('Ctrl Pts',(-0.0156493021159325,0.448583114629035,
-0.0506370131273639));
#34657=CARTESIAN_POINT('Ctrl Pts',(-0.382972295244705,0.234027977475628,
-0.0388535774797655));
#34658=CARTESIAN_POINT('Ctrl Pts',(-0.406288927791635,-0.190409270605048,
-0.0270701418321671));
#34659=CARTESIAN_POINT('Ctrl Pts',(-0.065075563863559,-0.44435965223454,
-0.0152867061845687));
#34660=CARTESIAN_POINT('Ctrl Pts',(0.33511883572153,-0.298373170952479,
-0.00350327053697042));
#34661=CARTESIAN_POINT('Ctrl Pts',(0.400447658493562,-0.0238667621989916,
0.00435235322809503));
#34662=CARTESIAN_POINT('Ctrl Pts',(0.368410545312071,0.09736079039141,0.00828016511062779));
#34663=CARTESIAN_POINT('Ctrl Pts',(0.353261248356923,0.0984256268479901,
-0.808280165110628));
#34664=CARTESIAN_POINT('Ctrl Pts',(0.320873744777592,0.214668218457478,
-0.804352353228095));
#34665=CARTESIAN_POINT('Ctrl Pts',(0.133061222988888,0.410799604104149,
-0.796496729463029));
#34666=CARTESIAN_POINT('Ctrl Pts',(-0.270250328453335,0.337281758900395,
-0.784713293815432));
#34667=CARTESIAN_POINT('Ctrl Pts',(-0.429987240670946,-0.0395996356841706,
-0.772929858167832));
#34668=CARTESIAN_POINT('Ctrl Pts',(-0.204102807690819,-0.380659338232164,
-0.761146422520236));
#34669=CARTESIAN_POINT('Ctrl Pts',(0.205280500560773,-0.380067979680208,
-0.749362986872634));
#34670=CARTESIAN_POINT('Ctrl Pts',(0.430221004412505,-0.03814614496241,
-0.73757955122504));
#34671=CARTESIAN_POINT('Ctrl Pts',(0.268936355313078,0.337988849201413,
-0.725796115577439));
#34672=CARTESIAN_POINT('Ctrl Pts',(-0.133856816475507,0.410667679452654,
-0.714012679929842));
#34673=CARTESIAN_POINT('Ctrl Pts',(-0.416443867536837,0.114602815262176,
-0.702229244282243));
#34674=CARTESIAN_POINT('Ctrl Pts',(-0.325120505661874,-0.284357059499448,
-0.690445808634644));
#34675=CARTESIAN_POINT('Ctrl Pts',(0.0581293370875048,-0.42799914074404,
-0.678662372987047));
#34676=CARTESIAN_POINT('Ctrl Pts',(0.389183031795877,-0.18734469165481,
-0.666878937339448));
#34677=CARTESIAN_POINT('Ctrl Pts',(0.370795509004288,0.221523423925956,
-0.655095501691849));
#34678=CARTESIAN_POINT('Ctrl Pts',(0.01947466339482,0.431488848993628,-0.643312066044252));
#34679=CARTESIAN_POINT('Ctrl Pts',(-0.349331872442684,0.254025649461116,
-0.631528630396653));
#34680=CARTESIAN_POINT('Ctrl Pts',(-0.404477903664755,-0.151523875264942,
-0.619745194749054));
#34681=CARTESIAN_POINT('Ctrl Pts',(-0.0964482111172401,-0.421022075925132,
-0.607961759101457));
#34682=CARTESIAN_POINT('Ctrl Pts',(0.298181065093639,-0.312489818103648,
-0.596178323453857));
#34683=CARTESIAN_POINT('Ctrl Pts',(0.425077339717431,0.0766231021527936,
-0.58439488780626));
#34684=CARTESIAN_POINT('Ctrl Pts',(0.170302001642169,0.396937110805389,
-0.57261145215866));
#34685=CARTESIAN_POINT('Ctrl Pts',(-0.237385354806005,0.360846274428439,
-0.560828016511064));
#34686=CARTESIAN_POINT('Ctrl Pts',(-0.431927390012499,0.000756107852782039,
-0.549044580863464));
#34687=CARTESIAN_POINT('Ctrl Pts',(-0.23864725077649,-0.360012959653721,
-0.537261145215866));
#34688=CARTESIAN_POINT('Ctrl Pts',(0.168911253077617,-0.397530916905416,
-0.525477709568268));
#34689=CARTESIAN_POINT('Ctrl Pts',(0.424806467266128,-0.0781108627956866,
-0.513694273920669));
#34690=CARTESIAN_POINT('Ctrl Pts',(0.299273295767665,0.31144395301484,-0.501910838273072));
#34691=CARTESIAN_POINT('Ctrl Pts',(-0.09497360474911,0.421357159456029,
-0.490127402625472));
#34692=CARTESIAN_POINT('Ctrl Pts',(-0.403944899851534,0.152939070662619,
-0.478343966977875));
#34693=CARTESIAN_POINT('Ctrl Pts',(-0.350219148585202,-0.252801086629681,
-0.466560531330277));
#34694=CARTESIAN_POINT('Ctrl Pts',(0.0179639724773354,-0.431554326974609,
-0.454777095682677));
#34695=CARTESIAN_POINT('Ctrl Pts',(0.370017468545135,-0.222820363550088,
-0.44299366003508));
#34696=CARTESIAN_POINT('Ctrl Pts',(0.389836932242896,0.185981202540365,
-0.431210224387481));
#34697=CARTESIAN_POINT('Ctrl Pts',(0.0596267163379231,0.427792585417331,
-0.419426788739883));
#34698=CARTESIAN_POINT('Ctrl Pts',(-0.32412157841533,0.285494384962672,
-0.407643353092284));
#34699=CARTESIAN_POINT('Ctrl Pts',(-0.416845183450903,-0.113145633910614,
-0.395859917444687));
#34700=CARTESIAN_POINT('Ctrl Pts',(-0.135288739726473,-0.410193610802121,
-0.384076481797087));
#34701=CARTESIAN_POINT('Ctrl Pts',(0.26774176226273,-0.338933902375868,
-0.37229304614949));
#34702=CARTESIAN_POINT('Ctrl Pts',(0.43037030253124,0.036650295197742,-0.360509610501891));
#34703=CARTESIAN_POINT('Ctrl Pts',(0.206574759685087,0.379326653561534,
-0.348726174854293));
#34704=CARTESIAN_POINT('Ctrl Pts',(-0.202701662390712,0.381410379383828,
-0.336942739206695));
#34705=CARTESIAN_POINT('Ctrl Pts',(-0.42997481059359,0.0410305214675364,
-0.325159303559096));
#34706=CARTESIAN_POINT('Ctrl Pts',(-0.271178982930367,-0.336190125774187,
-0.313375867911498));
#34707=CARTESIAN_POINT('Ctrl Pts',(0.131105043693952,-0.411549886334452,
-0.301592432263899));
#34708=CARTESIAN_POINT('Ctrl Pts',(0.415671500069678,-0.11738417891255,
-0.289808996616301));
#34709=CARTESIAN_POINT('Ctrl Pts',(0.3270117433223,0.28217930690808,-0.278025560968703));
#34710=CARTESIAN_POINT('Ctrl Pts',(-0.0552677460379093,0.428377540914321,
-0.266242125321104));
#34711=CARTESIAN_POINT('Ctrl Pts',(-0.387923020853791,0.189940967970258,
-0.254458689673507));
#34712=CARTESIAN_POINT('Ctrl Pts',(-0.372267093645615,-0.219041212858999,
-0.242675254025908));
#34713=CARTESIAN_POINT('Ctrl Pts',(-0.0223572228146897,-0.431349040839633,
-0.23089181837831));
#34714=CARTESIAN_POINT('Ctrl Pts',(0.347626915027303,-0.256353992842826,
-0.219108382730711));
#34715=CARTESIAN_POINT('Ctrl Pts',(0.405481221232114,0.148818089467912,
-0.207324947083113));
#34716=CARTESIAN_POINT('Ctrl Pts',(0.099259029312377,0.420368266046324,
-0.195541511435514));
#34717=CARTESIAN_POINT('Ctrl Pts',(-0.296086581363351,0.314475089920628,
-0.183758075787916));
#34718=CARTESIAN_POINT('Ctrl Pts',(-0.425579803407861,-0.073781367970967,
-0.171974640140318));
#34719=CARTESIAN_POINT('Ctrl Pts',(-0.172950214423107,-0.395790362464088,
-0.160191204492719));
#34720=CARTESIAN_POINT('Ctrl Pts',(0.234969088792759,-0.362424359876772,
-0.148407768845121));
#34721=CARTESIAN_POINT('Ctrl Pts',(0.431912809219259,-0.00364171360166344,
-0.136624333197522));
#34722=CARTESIAN_POINT('Ctrl Pts',(0.24104705268094,0.358410078154757,-0.124840897549924));
#34723=CARTESIAN_POINT('Ctrl Pts',(-0.16625106393219,0.398651311360297,
-0.113057461902326));
#34724=CARTESIAN_POINT('Ctrl Pts',(-0.424275888201981,0.0809459769193339,
-0.101274026254728));
#34725=CARTESIAN_POINT('Ctrl Pts',(-0.301345961598879,-0.309434825937711,
-0.0894905906071294));
#34726=CARTESIAN_POINT('Ctrl Pts',(0.092153430219589,-0.421987364221666,
-0.077707154959531));
#34727=CARTESIAN_POINT('Ctrl Pts',(0.402919513068942,-0.155624841789045,
-0.0659237193119326));
#34728=CARTESIAN_POINT('Ctrl Pts',(0.351889938005496,0.250437043074074,
-0.0541402836643342));
#34729=CARTESIAN_POINT('Ctrl Pts',(-0.0150603186063758,0.431700057785669,
-0.042356848016736));
#34730=CARTESIAN_POINT('Ctrl Pts',(-0.368558593927843,0.225220005178395,
-0.0305734123691377));
#34731=CARTESIAN_POINT('Ctrl Pts',(-0.390997672193642,-0.183242949728733,
-0.0187899767215392));
#34732=CARTESIAN_POINT('Ctrl Pts',(-0.0626263534318833,-0.427635551342383,
-0.00700654107394084));
#34733=CARTESIAN_POINT('Ctrl Pts',(0.322506166701548,-0.28714347674098,
0.00477689457365751));
#34734=CARTESIAN_POINT('Ctrl Pts',(0.385376247286455,-0.0229685030141659,
0.0126325183387229));
#34735=CARTESIAN_POINT('Ctrl Pts',(0.354544895947755,0.0936964800219656,
0.0165603302212557));
#34736=CARTESIAN_POINT('Ctrl Pts',(0.339445800272064,0.094576367569588,
-0.8));
#34737=CARTESIAN_POINT('Ctrl Pts',(0.308324917009509,0.206272908636879,
-0.796072188117467));
#34738=CARTESIAN_POINT('Ctrl Pts',(0.12785742430771,0.394733928544834,-0.788216564352402));
#34739=CARTESIAN_POINT('Ctrl Pts',(-0.259681296610673,0.32409124153759,
-0.776433128704804));
#34740=CARTESIAN_POINT('Ctrl Pts',(-0.413171169198995,-0.0380509611167842,
-0.764649693057206));
#34741=CARTESIAN_POINT('Ctrl Pts',(-0.196120693160165,-0.365772397335523,
-0.752866257409607));
#34742=CARTESIAN_POINT('Ctrl Pts',(0.197252328460035,-0.365204165813244,
-0.741082821762008));
#34743=CARTESIAN_POINT('Ctrl Pts',(0.413395790837222,-0.036654313951176,
-0.72929938611441));
#34744=CARTESIAN_POINT('Ctrl Pts',(0.258418710730661,0.324770678736576,
-0.717515950466812));
#34745=CARTESIAN_POINT('Ctrl Pts',(-0.128621903482862,0.394607163242637,
-0.705732514819214));
#34746=CARTESIAN_POINT('Ctrl Pts',(-0.400157454410652,0.110120893590899,
-0.693949079171615));
#34747=CARTESIAN_POINT('Ctrl Pts',(-0.312405594280605,-0.273236337338868,
-0.682165643524017));
#34748=CARTESIAN_POINT('Ctrl Pts',(0.055855997335481,-0.411260820487245,
-0.670382207876418));
#34749=CARTESIAN_POINT('Ctrl Pts',(0.373962743705146,-0.180017958610726,
-0.65859877222882));
#34750=CARTESIAN_POINT('Ctrl Pts',(0.356294325733907,0.212860018649936,
-0.646815336581221));
#34751=CARTESIAN_POINT('Ctrl Pts',(0.0187130423499051,0.414614052167785,
-0.635031900933623));
#34752=CARTESIAN_POINT('Ctrl Pts',(-0.335670095583304,0.244091137287262,
-0.623248465286025));
#34753=CARTESIAN_POINT('Ctrl Pts',(-0.388659459084311,-0.145598033576742,
-0.611465029638427));
#34754=CARTESIAN_POINT('Ctrl Pts',(-0.0926762852132086,-0.404556616836208,
-0.599681593990828));
#34755=CARTESIAN_POINT('Ctrl Pts',(0.286519709527895,-0.300268871483724,
-0.58789815834323));
#34756=CARTESIAN_POINT('Ctrl Pts',(0.408453286141698,0.0736265026253448,
-0.576114722695632));
#34757=CARTESIAN_POINT('Ctrl Pts',(0.163641779290076,0.381413573840065,
-0.564331287048033));
#34758=CARTESIAN_POINT('Ctrl Pts',(-0.228101616324409,0.34673418884258,
-0.552547851400434));
#34759=CARTESIAN_POINT('Ctrl Pts',(-0.415035442591431,0.000726537757461266,
-0.540764415752838));
#34760=CARTESIAN_POINT('Ctrl Pts',(-0.229314161684403,-0.34593346359491,
-0.528980980105238));
#34761=CARTESIAN_POINT('Ctrl Pts',(0.162305420542359,-0.381984157190963,
-0.517197544457641));
#34762=CARTESIAN_POINT('Ctrl Pts',(0.408193007052407,-0.0750560794736075,
-0.505414108810041));
#34763=CARTESIAN_POINT('Ctrl Pts',(0.287569224913323,0.299263908404139,
-0.493630673162444));
#34764=CARTESIAN_POINT('Ctrl Pts',(-0.09125934819834,0.40487859581871,-0.481847237514845));
#34765=CARTESIAN_POINT('Ctrl Pts',(-0.388147300145938,0.146957883083416,
-0.470063801867247));
#34766=CARTESIAN_POINT('Ctrl Pts',(-0.336522671861229,-0.242914465030589,
-0.458280366219648));
#34767=CARTESIAN_POINT('Ctrl Pts',(0.0172614319911864,-0.414676969416019,
-0.44649693057205));
#34768=CARTESIAN_POINT('Ctrl Pts',(0.355546713117099,-0.214106237165738,
-0.434713494924451));
#34769=CARTESIAN_POINT('Ctrl Pts',(0.37459107121508,0.178707793242271,-0.422930059276854));
#34770=CARTESIAN_POINT('Ctrl Pts',(0.0572948166238478,0.411062343188925,
-0.411146623629255));
#34771=CARTESIAN_POINT('Ctrl Pts',(-0.311445733383908,0.274329183932795,
-0.399363187981657));
#34772=CARTESIAN_POINT('Ctrl Pts',(-0.400543075540186,-0.108720700129763,
-0.387579752334058));
#34773=CARTESIAN_POINT('Ctrl Pts',(-0.129997826644863,-0.394151634612728,
-0.37579631668646));
#34774=CARTESIAN_POINT('Ctrl Pts',(0.257270836187783,-0.325678772484742,
-0.364012881038862));
#34775=CARTESIAN_POINT('Ctrl Pts',(0.41353925015983,0.0352169643329669,
-0.352229445391263));
#34776=CARTESIAN_POINT('Ctrl Pts',(0.198495971305819,0.364491831701348,
-0.340446009743665));
#34777=CARTESIAN_POINT('Ctrl Pts',(-0.194774344275583,0.366494066541952,
-0.328662574096066));
#34778=CARTESIAN_POINT('Ctrl Pts',(-0.413159225240875,0.0394258873847827,
-0.316879138448469));
#34779=CARTESIAN_POINT('Ctrl Pts',(-0.26057363298665,-0.323042300330899,
-0.30509570280087));
#34780=CARTESIAN_POINT('Ctrl Pts',(0.125977747866173,-0.395454868510028,
-0.293312267153272));
#34781=CARTESIAN_POINT('Ctrl Pts',(0.399415292924746,-0.112793482827731,
-0.281528831505673));
#34782=CARTESIAN_POINT('Ctrl Pts',(0.314222868844781,0.271143752956601,
-0.269745395858075));
#34783=CARTESIAN_POINT('Ctrl Pts',(-0.0531063182568973,0.411624422068856,
-0.257961960210477));
#34784=CARTESIAN_POINT('Ctrl Pts',(-0.372752009653287,0.182512698964285,
-0.246178524562878));
#34785=CARTESIAN_POINT('Ctrl Pts',(-0.357708359196582,-0.210474882646521,
-0.23439508891528));
#34786=CARTESIAN_POINT('Ctrl Pts',(-0.0214828697613762,-0.414479711673496,
-0.222611653267681));
#34787=CARTESIAN_POINT('Ctrl Pts',(0.334031816159831,-0.24632842310955,
-0.210828217620083));
#34788=CARTESIAN_POINT('Ctrl Pts',(0.389623538603825,0.142998066471633,
-0.199044781972485));
#34789=CARTESIAN_POINT('Ctrl Pts',(0.095377177077531,0.403928376352516,
-0.187261346324887));
#34790=CARTESIAN_POINT('Ctrl Pts',(-0.284507137502825,0.302176502688127,
-0.175477910677288));
#34791=CARTESIAN_POINT('Ctrl Pts',(-0.408936099329668,-0.0708959038461205,
-0.16369447502969));
#34792=CARTESIAN_POINT('Ctrl Pts',(-0.166186424962074,-0.380311672880833,
-0.151911039382091));
#34793=CARTESIAN_POINT('Ctrl Pts',(0.225779846375536,-0.348250558046386,
-0.140127603734493));
#34794=CARTESIAN_POINT('Ctrl Pts',(0.415021432028277,-0.00349929236118479,
-0.128344168086895));
#34795=CARTESIAN_POINT('Ctrl Pts',(0.231620111407843,0.344393268071943,
-0.116560732439296));
#34796=CARTESIAN_POINT('Ctrl Pts',(-0.159749266881169,0.383060734919559,
-0.104777296791698));
#34797=CARTESIAN_POINT('Ctrl Pts',(-0.407683178035285,0.0777803170938962,
-0.0929938611440997));
#34798=CARTESIAN_POINT('Ctrl Pts',(-0.289560832300336,-0.297333354878338,
-0.0812104254965016));
#34799=CARTESIAN_POINT('Ctrl Pts',(0.0885494659099983,-0.405484154345161,
-0.0694269898489031));
#34800=CARTESIAN_POINT('Ctrl Pts',(0.387162014500754,-0.149538618257732,
-0.0576435542013047));
#34801=CARTESIAN_POINT('Ctrl Pts',(0.338128119541936,0.240642875207636,
-0.0458601185537062));
#34802=CARTESIAN_POINT('Ctrl Pts',(-0.01447133509682,0.414817000942304,
-0.0340766829061081));
#34803=CARTESIAN_POINT('Ctrl Pts',(-0.354144892610982,0.216412032881162,
-0.0222932472585097));
#34804=CARTESIAN_POINT('Ctrl Pts',(-0.375706416595649,-0.176076628852418,
-0.0105098116109113));
#34805=CARTESIAN_POINT('Ctrl Pts',(-0.0601771430002081,-0.410911450450226,
0.00127362403668707));
#34806=CARTESIAN_POINT('Ctrl Pts',(0.309893497681566,-0.27591378252948,
0.0130570596842854));
#34807=CARTESIAN_POINT('Ctrl Pts',(0.370304836079347,-0.0220702438293411,
0.0209126834493508));
#34808=CARTESIAN_POINT('Ctrl Pts',(0.340679246583439,0.0900321696525211,
0.0248404953318836));
#34809=CARTESIAN_POINT('',(0.382276194676387,0.101025100760854,-1.11022302462516E-16));
#34810=CARTESIAN_POINT('Ctrl Pts',(-0.0877607245812972,-0.341761560210009,
-9.71445146547012E-17));
#34811=CARTESIAN_POINT('Ctrl Pts',(-0.0758129511624255,-0.345685911786213,
-1.177492375083E-16));
#34812=CARTESIAN_POINT('Ctrl Pts',(-0.0636801234265344,-0.348930529057438,
-1.71071818152792E-16));
#34813=CARTESIAN_POINT('Ctrl Pts',(-0.0514067357749123,-0.351459262350156,
-7.97972798949331E-17));
#34814=CARTESIAN_POINT('Ctrl Pts',(-0.0333136723076778,-0.355187045848529,
5.12874859358975E-17));
#34815=CARTESIAN_POINT('Ctrl Pts',(-0.0149152850678594,-0.357361071442325,
-9.16194412763928E-17));
#34816=CARTESIAN_POINT('Ctrl Pts',(0.0036226861155836,-0.358060875566304,
-2.67147415300428E-16));
#34817=CARTESIAN_POINT('Ctrl Pts',(0.00988803044492662,-0.35829739086544,
-3.26471231580539E-16));
#34818=CARTESIAN_POINT('Ctrl Pts',(0.0161593613325987,-0.358364790839047,
2.4941399093868E-17));
#34819=CARTESIAN_POINT('Ctrl Pts',(0.0224287212483521,-0.35826689462958,
2.42861286636753E-17));
#34820=CARTESIAN_POINT('Ctrl Pts',(0.0394302907234294,-0.358001414703562,
2.25091329426463E-17));
#34821=CARTESIAN_POINT('Ctrl Pts',(0.056420623703811,-0.356522253769826,
-2.5213610675368E-16));
#34822=CARTESIAN_POINT('Ctrl Pts',(0.0732737027369599,-0.353889163118092,
-2.70616862252382E-16));
#34823=CARTESIAN_POINT('Ctrl Pts',(0.080079917994765,-0.352825773945481,
-2.7808042424029E-16));
#34824=CARTESIAN_POINT('Ctrl Pts',(0.0868637834211038,-0.351573895775077,
1.10500851824191E-16));
#34825=CARTESIAN_POINT('Ctrl Pts',(0.093617012145756,-0.3501363439148,1.31838984174237E-16));
#34826=CARTESIAN_POINT('Ctrl Pts',(0.0991248085493264,-0.348963905768721,
1.49241932217071E-16));
#34827=CARTESIAN_POINT('Ctrl Pts',(0.104611759658228,-0.347667843483011,
-2.60939886659057E-16));
#34828=CARTESIAN_POINT('Ctrl Pts',(0.110060136668145,-0.346253488087783,
-2.70616862252382E-16));
#34829=CARTESIAN_POINT('Ctrl Pts',(0.130533905168791,-0.340938660408493,
-3.06980747813803E-16));
#34830=CARTESIAN_POINT('Ctrl Pts',(0.150511485695683,-0.333947922137602,
-1.0781477527908E-16));
#34831=CARTESIAN_POINT('Ctrl Pts',(0.169762335881931,-0.325386261459349,
-2.77555756156289E-17));
#34832=CARTESIAN_POINT('Ctrl Pts',(0.18344782334648,-0.319299751058283,
2.91587509110359E-17));
#34833=CARTESIAN_POINT('Ctrl Pts',(0.196766296793287,-0.312418138560091,
1.39805396323208E-17));
#34834=CARTESIAN_POINT('Ctrl Pts',(0.209631272392485,-0.304763602083614,
3.81639164714898E-17));
#34835=CARTESIAN_POINT('Ctrl Pts',(0.215617622250039,-0.301201781620584,
4.9416961872163E-17));
#34836=CARTESIAN_POINT('Ctrl Pts',(0.221505701159809,-0.29747243078369,
7.35255697550562E-18));
#34837=CARTESIAN_POINT('Ctrl Pts',(0.227286255175715,-0.29357690861442,
1.04083408558608E-17));
#34838=CARTESIAN_POINT('Ctrl Pts',(0.231373893127996,-0.290822244577161,
1.25691957028073E-17));
#34839=CARTESIAN_POINT('Ctrl Pts',(0.235404366734835,-0.287986626798667,
-6.88599098182481E-17));
#34840=CARTESIAN_POINT('Ctrl Pts',(0.239368194670903,-0.285075849963472,
-7.11236625150491E-17));
#34841=CARTESIAN_POINT('Ctrl Pts',(0.253900448925098,-0.274404309793586,
-7.94230716440859E-17));
#34842=CARTESIAN_POINT('Ctrl Pts',(0.267564666409036,-0.262706457293931,
1.34449454094602E-16));
#34843=CARTESIAN_POINT('Ctrl Pts',(0.280217681766689,-0.250031803400258,
7.45931094670027E-17));
#34844=CARTESIAN_POINT('Ctrl Pts',(0.291337752368455,-0.238892715825742,
2.51264174834658E-17));
#34845=CARTESIAN_POINT('Ctrl Pts',(0.301677019629086,-0.226998713289539,
-1.40107180888897E-16));
#34846=CARTESIAN_POINT('Ctrl Pts',(0.311222774198572,-0.214447092320648,
-1.78676518025611E-16));
#34847=CARTESIAN_POINT('Ctrl Pts',(0.315932140355436,-0.208254792008042,
-1.97704571772661E-16));
#34848=CARTESIAN_POINT('Ctrl Pts',(0.320448187331642,-0.201902232686996,
-1.19650750174349E-16));
#34849=CARTESIAN_POINT('Ctrl Pts',(0.324768233576707,-0.195400111602237,
-1.37043154602168E-16));
#34850=CARTESIAN_POINT('Ctrl Pts',(0.328357743214907,-0.189997524458835,
-1.51494435857885E-16));
#34851=CARTESIAN_POINT('Ctrl Pts',(0.331813146917509,-0.184489067659585,
-9.43126563239188E-17));
#34852=CARTESIAN_POINT('Ctrl Pts',(0.335120725151517,-0.178902066827157,
-7.63278329429795E-17));
#34853=CARTESIAN_POINT('Ctrl Pts',(0.345962373971419,-0.160588879142313,
-1.73768043084045E-17));
#34854=CARTESIAN_POINT('Ctrl Pts',(0.355249503471015,-0.141391317035762,
-5.63017718245087E-17));
#34855=CARTESIAN_POINT('Ctrl Pts',(0.362958797935917,-0.121547298462339,
8.67361737988404E-19));
#34856=CARTESIAN_POINT('Ctrl Pts',(0.369776633578432,-0.103997928966007,
5.14257829046096E-17));
#34857=CARTESIAN_POINT('Ctrl Pts',(0.375360154194583,-0.0859417157175588,
-5.76413480178255E-17));
#34858=CARTESIAN_POINT('Ctrl Pts',(0.379665889922516,-0.0675259946344044,
-9.4542429440736E-17));
#34859=CARTESIAN_POINT('Ctrl Pts',(0.380989312850641,-0.0618656873003285,
-1.05884448624796E-16));
#34860=CARTESIAN_POINT('Ctrl Pts',(0.382191821778051,-0.0561713465087971,
-2.82818896685015E-16));
#34861=CARTESIAN_POINT('Ctrl Pts',(0.383271604327089,-0.0504471153025764,
-3.25260651745651E-16));
#34862=CARTESIAN_POINT('Ctrl Pts',(0.384221568788495,-0.0454110863172686,
-3.62599798431484E-16));
#34863=CARTESIAN_POINT('Ctrl Pts',(0.385074753570206,-0.0403613371122496,
2.29496281791598E-18));
#34864=CARTESIAN_POINT('Ctrl Pts',(0.385830757252302,-0.0353015274382432,
4.33680868994202E-18));
#34865=CARTESIAN_POINT('Ctrl Pts',(0.389216753731649,-0.0126396037623478,
1.34818473951543E-17));
#34866=CARTESIAN_POINT('Ctrl Pts',(0.390658467045214,0.0102261533125763,
-1.65967614351841E-16));
#34867=CARTESIAN_POINT('Ctrl Pts',(0.390095953236443,0.0330330050049388,
-2.19008838842072E-16));
#34868=CARTESIAN_POINT('Ctrl Pts',(0.389567451361758,0.0544608591964589,
-2.68842969385262E-16));
#34869=CARTESIAN_POINT('Ctrl Pts',(0.387269745794741,0.0758382323114046,
-4.68604663216744E-18));
#34870=CARTESIAN_POINT('Ctrl Pts',(0.38310379834931,0.0969520739608447,
1.7130394325271E-17));
#34871=CARTESIAN_POINT('Ctrl Pts',(0.38283569725694,0.0983108630681218,
1.8534399471502E-17));
#34872=CARTESIAN_POINT('Ctrl Pts',(0.382559840678217,0.0996685580786185,
-1.11708830315621E-16));
#34873=CARTESIAN_POINT('Ctrl Pts',(0.382276194676387,0.101025100760854,
-1.12757025938492E-16));
#34874=CARTESIAN_POINT('Ctrl Pts',(0.382276194676389,0.101025100760849,
-2.50371428041207E-16));
#34875=CARTESIAN_POINT('Ctrl Pts',(0.415519069700669,-0.0247650213838198,
-0.00392781188253294));
#34876=CARTESIAN_POINT('Ctrl Pts',(0.381625287221089,-0.1671839432739,-0.00785562376506566));
#34877=CARTESIAN_POINT('Ctrl Pts',(0.295469016141844,-0.263640218879391,
-0.0117834356475983));
#34878=CARTESIAN_POINT('Ctrl Pts',(0.209312745062596,-0.360096494484885,
-0.0157112475301311));
#34879=CARTESIAN_POINT('Ctrl Pts',(0.0708939853836822,-0.41059012380579,
-0.0196390594126638));
#34880=CARTESIAN_POINT('Ctrl Pts',(-0.0573246293048418,-0.391918911525354,
-0.0235668712951966));
#34881=CARTESIAN_POINT('Ctrl Pts',(-0.185543243993364,-0.373247699244919,
-0.0274946831777294));
#34882=CARTESIAN_POINT('Ctrl Pts',(-0.303561713691496,-0.285411645363141,
-0.0314224950602622));
#34883=CARTESIAN_POINT('Ctrl Pts',(-0.358538584069218,-0.168091694879883,
-0.0353503069427949));
#34884=CARTESIAN_POINT('Ctrl Pts',(-0.382957007318537,-0.115983086535923,
-0.0370948764741711));
#34885=CARTESIAN_POINT('Ctrl Pts',(-0.394938808705564,-0.058058000231184,
-0.0388394460055472));
#34886=CARTESIAN_POINT('Ctrl Pts',(-0.394794988713166,-8.02750947288822E-5,
-0.0405840155369234));
#34887=CARTESIAN_POINT('Origin',(-0.5,0.5,0.1));
#34888=CARTESIAN_POINT('',(-0.58,0.5,0.));
#34889=CARTESIAN_POINT('Origin',(-0.5,0.5,0.));
#34890=CARTESIAN_POINT('',(-0.58,0.5,0.2));
#34891=CARTESIAN_POINT('',(-0.58,0.5,0.1));
#34892=CARTESIAN_POINT('Origin',(-0.5,0.5,0.2));
#34893=CARTESIAN_POINT('Origin',(0.5,0.5,0.1));
#34894=CARTESIAN_POINT('',(0.42,0.5,0.));
#34895=CARTESIAN_POINT('Origin',(0.5,0.5,0.));
#34896=CARTESIAN_POINT('',(0.42,0.5,0.2));
#34897=CARTESIAN_POINT('',(0.42,0.5,0.1));
#34898=CARTESIAN_POINT('Origin',(0.5,0.5,0.2));
#34899=CARTESIAN_POINT('Origin',(0.5,-0.5,0.1));
#34900=CARTESIAN_POINT('',(0.42,-0.5,0.));
#34901=CARTESIAN_POINT('Origin',(0.5,-0.5,0.));
#34902=CARTESIAN_POINT('',(0.42,-0.5,0.2));
#34903=CARTESIAN_POINT('',(0.42,-0.5,0.1));
#34904=CARTESIAN_POINT('Origin',(0.5,-0.5,0.2));
#34905=CARTESIAN_POINT('Origin',(-0.5,-0.5,0.1));
#34906=CARTESIAN_POINT('',(-0.58,-0.5,0.));
#34907=CARTESIAN_POINT('Origin',(-0.5,-0.5,0.));
#34908=CARTESIAN_POINT('',(-0.58,-0.5,0.2));
#34909=CARTESIAN_POINT('',(-0.58,-0.5,0.1));
#34910=CARTESIAN_POINT('Origin',(-0.5,-0.5,0.2));
#34911=CARTESIAN_POINT('Origin',(0.463644396618753,-0.12423314164921,0.66));
#34912=CARTESIAN_POINT('',(0.479742226065207,-0.140880788363777,0.66));
#34913=CARTESIAN_POINT('',(0.479742226065207,-0.140880788363777,1.34));
#34914=CARTESIAN_POINT('',(0.479742226065207,-0.140880788363777,1.));
#34915=CARTESIAN_POINT('',(0.463644396618753,-0.12423314164921,0.66));
#34916=CARTESIAN_POINT('',(0.463644396618753,-0.12423314164921,0.66));
#34917=CARTESIAN_POINT('',(0.463644396618753,-0.12423314164921,1.34));
#34918=CARTESIAN_POINT('',(0.463644396618753,-0.12423314164921,0.66));
#34919=CARTESIAN_POINT('',(0.463644396618753,-0.12423314164921,1.34));
#34920=CARTESIAN_POINT('Origin',(0.492622171407425,-0.131997713002286,1.34));
#34921=CARTESIAN_POINT('',(0.485909349222455,-0.117864771404394,1.34));
#34922=CARTESIAN_POINT('Origin',(0.,0.,1.34));
#34923=CARTESIAN_POINT('',(0.530916762985404,-0.104991450732855,1.34));
#34924=CARTESIAN_POINT('Origin',(0.530916762985404,-0.104991450732855,0.66));
#34925=CARTESIAN_POINT('',(0.485909349222455,-0.117864771404394,0.66));
#34926=CARTESIAN_POINT('',(0.485909349222455,-0.117864771404394,1.));
#34927=CARTESIAN_POINT('',(0.530916762985404,-0.104991450732855,0.66));
#34928=CARTESIAN_POINT('Origin',(0.492622171407425,-0.131997713002286,0.66));
#34929=CARTESIAN_POINT('Origin',(0.,0.,0.66));
#34930=CARTESIAN_POINT('Origin',(0.41569219381653,-0.24,0.66));
#34931=CARTESIAN_POINT('',(0.42693277500019,-0.260246816754091,0.66));
#34932=CARTESIAN_POINT('',(0.42693277500019,-0.260246816754091,1.34));
#34933=CARTESIAN_POINT('',(0.42693277500019,-0.260246816754091,1.));
#34934=CARTESIAN_POINT('',(0.41569219381653,-0.24,0.66));
#34935=CARTESIAN_POINT('',(0.41569219381653,-0.24,0.66));
#34936=CARTESIAN_POINT('',(0.41569219381653,-0.24,1.34));
#34937=CARTESIAN_POINT('',(0.41569219381653,-0.24,0.66));
#34938=CARTESIAN_POINT('',(0.41569219381653,-0.24,1.34));
#34939=CARTESIAN_POINT('Origin',(0.441672955930064,-0.255,1.34));
#34940=CARTESIAN_POINT('',(0.438846742063171,-0.239611220481305,1.34));
#34941=CARTESIAN_POINT('Origin',(0.,0.,1.34));
#34942=CARTESIAN_POINT('',(0.485652425954788,-0.238825323427225,1.34));
#34943=CARTESIAN_POINT('Origin',(0.485652425954788,-0.238825323427225,0.66));
#34944=CARTESIAN_POINT('',(0.438846742063171,-0.239611220481305,0.66));
#34945=CARTESIAN_POINT('',(0.438846742063171,-0.239611220481305,1.));
#34946=CARTESIAN_POINT('',(0.485652425954788,-0.238825323427225,0.66));
#34947=CARTESIAN_POINT('Origin',(0.441672955930064,-0.255,0.66));
#34948=CARTESIAN_POINT('Origin',(0.,0.,0.66));
#34949=CARTESIAN_POINT('Origin',(0.339411254969543,-0.339411254969543,0.66));
#34950=CARTESIAN_POINT('',(0.345028560858678,-0.361877454660814,0.66));
#34951=CARTESIAN_POINT('',(0.345028560858678,-0.361877454660814,1.34));
#34952=CARTESIAN_POINT('',(0.345028560858678,-0.361877454660814,1.));
#34953=CARTESIAN_POINT('',(0.339411254969543,-0.339411254969543,0.66));
#34954=CARTESIAN_POINT('',(0.339411254969543,-0.339411254969543,0.66));
#34955=CARTESIAN_POINT('',(0.339411254969543,-0.339411254969543,1.34));
#34956=CARTESIAN_POINT('',(0.339411254969543,-0.339411254969543,0.66));
#34957=CARTESIAN_POINT('',(0.339411254969543,-0.339411254969543,1.34));
#34958=CARTESIAN_POINT('Origin',(0.360624458405139,-0.360624458405139,1.34));
#34959=CARTESIAN_POINT('',(0.361877454660813,-0.345028560858679,1.34));
#34960=CARTESIAN_POINT('Origin',(0.,0.,1.34));
#34961=CARTESIAN_POINT('',(0.407291678673935,-0.356383645007537,1.34));
#34962=CARTESIAN_POINT('Origin',(0.407291678673935,-0.356383645007537,0.66));
#34963=CARTESIAN_POINT('',(0.361877454660813,-0.345028560858679,0.66));
#34964=CARTESIAN_POINT('',(0.361877454660813,-0.345028560858679,1.));
#34965=CARTESIAN_POINT('',(0.407291678673935,-0.356383645007537,0.66));
#34966=CARTESIAN_POINT('Origin',(0.360624458405139,-0.360624458405139,0.66));
#34967=CARTESIAN_POINT('Origin',(0.,0.,0.66));
#34968=CARTESIAN_POINT('Origin',(0.24,-0.415692193816531,0.66));
#34969=CARTESIAN_POINT('',(0.239611220481304,-0.438846742063172,0.66));
#34970=CARTESIAN_POINT('',(0.239611220481304,-0.438846742063172,1.34));
#34971=CARTESIAN_POINT('',(0.239611220481304,-0.438846742063172,1.));
#34972=CARTESIAN_POINT('',(0.24,-0.415692193816531,0.66));
#34973=CARTESIAN_POINT('',(0.24,-0.415692193816531,0.66));
#34974=CARTESIAN_POINT('',(0.24,-0.415692193816531,1.34));
#34975=CARTESIAN_POINT('',(0.24,-0.415692193816531,0.66));
#34976=CARTESIAN_POINT('',(0.24,-0.415692193816531,1.34));
#34977=CARTESIAN_POINT('Origin',(0.255,-0.441672955930064,1.34));
#34978=CARTESIAN_POINT('',(0.260246816754091,-0.42693277500019,1.34));
#34979=CARTESIAN_POINT('Origin',(0.,0.,1.34));
#34980=CARTESIAN_POINT('',(0.301174676572775,-0.449655010132406,1.34));
#34981=CARTESIAN_POINT('Origin',(0.301174676572775,-0.449655010132406,0.66));
#34982=CARTESIAN_POINT('',(0.260246816754091,-0.42693277500019,0.66));
#34983=CARTESIAN_POINT('',(0.260246816754091,-0.42693277500019,1.));
#34984=CARTESIAN_POINT('',(0.301174676572775,-0.449655010132406,0.66));
#34985=CARTESIAN_POINT('Origin',(0.255,-0.441672955930064,0.66));
#34986=CARTESIAN_POINT('Origin',(0.,0.,0.66));
#34987=CARTESIAN_POINT('Origin',(0.12423314164921,-0.463644396618753,0.66));
#34988=CARTESIAN_POINT('',(0.117864771404394,-0.485909349222455,0.66));
#34989=CARTESIAN_POINT('',(0.117864771404394,-0.485909349222455,1.34));
#34990=CARTESIAN_POINT('',(0.117864771404394,-0.485909349222455,1.));
#34991=CARTESIAN_POINT('',(0.12423314164921,-0.463644396618753,0.66));
#34992=CARTESIAN_POINT('',(0.12423314164921,-0.463644396618753,0.66));
#34993=CARTESIAN_POINT('',(0.12423314164921,-0.463644396618753,1.34));
#34994=CARTESIAN_POINT('',(0.12423314164921,-0.463644396618753,0.66));
#34995=CARTESIAN_POINT('',(0.12423314164921,-0.463644396618753,1.34));
#34996=CARTESIAN_POINT('Origin',(0.131997713002285,-0.492622171407425,1.34));
#34997=CARTESIAN_POINT('',(0.140880788363777,-0.479742226065208,1.34));
#34998=CARTESIAN_POINT('Origin',(0.,0.,1.34));
#34999=CARTESIAN_POINT('',(0.174533117977867,-0.512283129406789,1.34));
#35000=CARTESIAN_POINT('Origin',(0.174533117977867,-0.512283129406789,0.66));
#35001=CARTESIAN_POINT('',(0.140880788363777,-0.479742226065208,0.66));
#35002=CARTESIAN_POINT('',(0.140880788363777,-0.479742226065208,1.));
#35003=CARTESIAN_POINT('',(0.174533117977867,-0.512283129406789,0.66));
#35004=CARTESIAN_POINT('Origin',(0.131997713002285,-0.492622171407425,0.66));
#35005=CARTESIAN_POINT('Origin',(0.,0.,0.66));
#35006=CARTESIAN_POINT('Origin',(-6.93889390390723E-17,-0.48,0.66));
#35007=CARTESIAN_POINT('',(-0.0119139670629818,-0.499858037235396,0.66));
#35008=CARTESIAN_POINT('',(-0.0119139670629818,-0.499858037235396,1.34));
#35009=CARTESIAN_POINT('',(-0.0119139670629818,-0.499858037235396,1.));
#35010=CARTESIAN_POINT('',(-6.93889390390723E-17,-0.48,0.66));
#35011=CARTESIAN_POINT('',(-6.93889390390723E-17,-0.48,0.66));
#35012=CARTESIAN_POINT('',(-6.93889390390723E-17,-0.48,1.34));
#35013=CARTESIAN_POINT('',(-6.93889390390723E-17,-0.48,0.66));
#35014=CARTESIAN_POINT('',(-6.93889390390723E-17,-0.48,1.34));
#35015=CARTESIAN_POINT('Origin',(-8.32667268468867E-17,-0.51,1.34));
#35016=CARTESIAN_POINT('',(0.0119139670629816,-0.499858037235396,1.34));
#35017=CARTESIAN_POINT('Origin',(0.,0.,1.34));
#35018=CARTESIAN_POINT('',(0.0359974158223829,-0.54,1.34));
#35019=CARTESIAN_POINT('Origin',(0.0359974158223829,-0.54,0.66));
#35020=CARTESIAN_POINT('',(0.0119139670629816,-0.499858037235396,0.66));
#35021=CARTESIAN_POINT('',(0.0119139670629816,-0.499858037235396,1.));
#35022=CARTESIAN_POINT('',(0.0359974158223829,-0.54,0.66));
#35023=CARTESIAN_POINT('Origin',(-8.32667268468867E-17,-0.51,0.66));
#35024=CARTESIAN_POINT('Origin',(0.,0.,0.66));
#35025=CARTESIAN_POINT('Origin',(-0.12423314164921,-0.463644396618753,0.66));
#35026=CARTESIAN_POINT('',(-0.140880788363777,-0.479742226065207,0.66));
#35027=CARTESIAN_POINT('',(-0.140880788363777,-0.479742226065207,1.34));
#35028=CARTESIAN_POINT('',(-0.140880788363777,-0.479742226065207,1.));
#35029=CARTESIAN_POINT('',(-0.12423314164921,-0.463644396618753,0.66));
#35030=CARTESIAN_POINT('',(-0.12423314164921,-0.463644396618753,0.66));
#35031=CARTESIAN_POINT('',(-0.12423314164921,-0.463644396618753,1.34));
#35032=CARTESIAN_POINT('',(-0.12423314164921,-0.463644396618753,0.66));
#35033=CARTESIAN_POINT('',(-0.12423314164921,-0.463644396618753,1.34));
#35034=CARTESIAN_POINT('Origin',(-0.131997713002286,-0.492622171407425,
1.34));
#35035=CARTESIAN_POINT('',(-0.117864771404394,-0.485909349222455,1.34));
#35036=CARTESIAN_POINT('Origin',(0.,0.,1.34));
#35037=CARTESIAN_POINT('',(-0.104991450732855,-0.530916762985404,1.34));
#35038=CARTESIAN_POINT('Origin',(-0.104991450732855,-0.530916762985404,
0.66));
#35039=CARTESIAN_POINT('',(-0.117864771404394,-0.485909349222455,0.66));
#35040=CARTESIAN_POINT('',(-0.117864771404394,-0.485909349222455,1.));
#35041=CARTESIAN_POINT('',(-0.104991450732855,-0.530916762985404,0.66));
#35042=CARTESIAN_POINT('Origin',(-0.131997713002286,-0.492622171407425,
0.66));
#35043=CARTESIAN_POINT('Origin',(0.,0.,0.66));
#35044=CARTESIAN_POINT('Origin',(-0.24,-0.41569219381653,0.66));
#35045=CARTESIAN_POINT('',(-0.260246816754091,-0.42693277500019,0.66));
#35046=CARTESIAN_POINT('',(-0.260246816754091,-0.42693277500019,1.34));
#35047=CARTESIAN_POINT('',(-0.260246816754091,-0.42693277500019,1.));
#35048=CARTESIAN_POINT('',(-0.24,-0.41569219381653,0.66));
#35049=CARTESIAN_POINT('',(-0.24,-0.41569219381653,0.66));
#35050=CARTESIAN_POINT('',(-0.24,-0.41569219381653,1.34));
#35051=CARTESIAN_POINT('',(-0.24,-0.41569219381653,0.66));
#35052=CARTESIAN_POINT('',(-0.24,-0.41569219381653,1.34));
#35053=CARTESIAN_POINT('Origin',(-0.255,-0.441672955930064,1.34));
#35054=CARTESIAN_POINT('',(-0.239611220481305,-0.438846742063171,1.34));
#35055=CARTESIAN_POINT('Origin',(0.,0.,1.34));
#35056=CARTESIAN_POINT('',(-0.238825323427225,-0.485652425954788,1.34));
#35057=CARTESIAN_POINT('Origin',(-0.238825323427225,-0.485652425954788,
0.66));
#35058=CARTESIAN_POINT('',(-0.239611220481305,-0.438846742063171,0.66));
#35059=CARTESIAN_POINT('',(-0.239611220481305,-0.438846742063171,1.));
#35060=CARTESIAN_POINT('',(-0.238825323427225,-0.485652425954788,0.66));
#35061=CARTESIAN_POINT('Origin',(-0.255,-0.441672955930064,0.66));
#35062=CARTESIAN_POINT('Origin',(0.,0.,0.66));
#35063=CARTESIAN_POINT('Origin',(-0.339411254969543,-0.339411254969543,
0.66));
#35064=CARTESIAN_POINT('',(-0.361877454660814,-0.345028560858678,0.66));
#35065=CARTESIAN_POINT('',(-0.361877454660814,-0.345028560858678,1.34));
#35066=CARTESIAN_POINT('',(-0.361877454660814,-0.345028560858678,1.));
#35067=CARTESIAN_POINT('',(-0.339411254969543,-0.339411254969543,0.66));
#35068=CARTESIAN_POINT('',(-0.339411254969543,-0.339411254969543,0.66));
#35069=CARTESIAN_POINT('',(-0.339411254969543,-0.339411254969543,1.34));
#35070=CARTESIAN_POINT('',(-0.339411254969543,-0.339411254969543,0.66));
#35071=CARTESIAN_POINT('',(-0.339411254969543,-0.339411254969543,1.34));
#35072=CARTESIAN_POINT('Origin',(-0.360624458405139,-0.360624458405139,
1.34));
#35073=CARTESIAN_POINT('',(-0.345028560858679,-0.361877454660813,1.34));
#35074=CARTESIAN_POINT('Origin',(0.,0.,1.34));
#35075=CARTESIAN_POINT('',(-0.356383645007537,-0.407291678673934,1.34));
#35076=CARTESIAN_POINT('Origin',(-0.356383645007537,-0.407291678673934,
0.66));
#35077=CARTESIAN_POINT('',(-0.345028560858679,-0.361877454660813,0.66));
#35078=CARTESIAN_POINT('',(-0.345028560858679,-0.361877454660813,1.));
#35079=CARTESIAN_POINT('',(-0.356383645007537,-0.407291678673934,0.66));
#35080=CARTESIAN_POINT('Origin',(-0.360624458405139,-0.360624458405139,
0.66));
#35081=CARTESIAN_POINT('Origin',(0.,0.,0.66));
#35082=CARTESIAN_POINT('Origin',(-0.415692193816531,-0.24,0.66));
#35083=CARTESIAN_POINT('',(-0.438846742063171,-0.239611220481304,0.66));
#35084=CARTESIAN_POINT('',(-0.438846742063171,-0.239611220481304,1.34));
#35085=CARTESIAN_POINT('',(-0.438846742063171,-0.239611220481304,1.));
#35086=CARTESIAN_POINT('',(-0.415692193816531,-0.24,0.66));
#35087=CARTESIAN_POINT('',(-0.415692193816531,-0.24,0.66));
#35088=CARTESIAN_POINT('',(-0.415692193816531,-0.24,1.34));
#35089=CARTESIAN_POINT('',(-0.415692193816531,-0.24,0.66));
#35090=CARTESIAN_POINT('',(-0.415692193816531,-0.24,1.34));
#35091=CARTESIAN_POINT('Origin',(-0.441672955930064,-0.255,1.34));
#35092=CARTESIAN_POINT('',(-0.42693277500019,-0.260246816754091,1.34));
#35093=CARTESIAN_POINT('Origin',(0.,0.,1.34));
#35094=CARTESIAN_POINT('',(-0.449655010132406,-0.301174676572776,1.34));
#35095=CARTESIAN_POINT('Origin',(-0.449655010132406,-0.301174676572776,
0.66));
#35096=CARTESIAN_POINT('',(-0.42693277500019,-0.260246816754091,0.66));
#35097=CARTESIAN_POINT('',(-0.42693277500019,-0.260246816754091,1.));
#35098=CARTESIAN_POINT('',(-0.449655010132406,-0.301174676572776,0.66));
#35099=CARTESIAN_POINT('Origin',(-0.441672955930064,-0.255,0.66));
#35100=CARTESIAN_POINT('Origin',(0.,0.,0.66));
#35101=CARTESIAN_POINT('Origin',(-0.463644396618753,-0.12423314164921,0.66));
#35102=CARTESIAN_POINT('',(-0.485909349222455,-0.117864771404394,0.66));
#35103=CARTESIAN_POINT('',(-0.485909349222455,-0.117864771404394,1.34));
#35104=CARTESIAN_POINT('',(-0.485909349222455,-0.117864771404394,1.));
#35105=CARTESIAN_POINT('',(-0.463644396618753,-0.12423314164921,0.66));
#35106=CARTESIAN_POINT('',(-0.463644396618753,-0.12423314164921,0.66));
#35107=CARTESIAN_POINT('',(-0.463644396618753,-0.12423314164921,1.34));
#35108=CARTESIAN_POINT('',(-0.463644396618753,-0.12423314164921,0.66));
#35109=CARTESIAN_POINT('',(-0.463644396618753,-0.12423314164921,1.34));
#35110=CARTESIAN_POINT('Origin',(-0.492622171407425,-0.131997713002285,
1.34));
#35111=CARTESIAN_POINT('',(-0.479742226065208,-0.140880788363777,1.34));
#35112=CARTESIAN_POINT('Origin',(0.,0.,1.34));
#35113=CARTESIAN_POINT('',(-0.512283129406789,-0.174533117977868,1.34));
#35114=CARTESIAN_POINT('Origin',(-0.512283129406789,-0.174533117977868,
0.66));
#35115=CARTESIAN_POINT('',(-0.479742226065208,-0.140880788363777,0.66));
#35116=CARTESIAN_POINT('',(-0.479742226065208,-0.140880788363777,1.));
#35117=CARTESIAN_POINT('',(-0.512283129406789,-0.174533117977868,0.66));
#35118=CARTESIAN_POINT('Origin',(-0.492622171407425,-0.131997713002285,
0.66));
#35119=CARTESIAN_POINT('Origin',(0.,0.,0.66));
#35120=CARTESIAN_POINT('Origin',(-0.48,5.55111512312578E-17,0.66));
#35121=CARTESIAN_POINT('',(-0.499858037235396,0.0119139670629818,0.66));
#35122=CARTESIAN_POINT('',(-0.499858037235396,0.0119139670629818,1.34));
#35123=CARTESIAN_POINT('',(-0.499858037235396,0.0119139670629818,1.));
#35124=CARTESIAN_POINT('',(-0.48,5.55111512312578E-17,0.66));
#35125=CARTESIAN_POINT('',(-0.48,5.55111512312578E-17,0.66));
#35126=CARTESIAN_POINT('',(-0.48,5.55111512312578E-17,1.34));
#35127=CARTESIAN_POINT('',(-0.48,5.55111512312578E-17,0.66));
#35128=CARTESIAN_POINT('',(-0.48,5.55111512312578E-17,1.34));
#35129=CARTESIAN_POINT('Origin',(-0.51,5.55111512312578E-17,1.34));
#35130=CARTESIAN_POINT('',(-0.5,-6.12323399573677E-17,1.34));
#35131=CARTESIAN_POINT('Origin',(0.,0.,1.34));
#35132=CARTESIAN_POINT('',(-0.499858037235396,-0.0119139670629816,1.34));
#35133=CARTESIAN_POINT('',(-0.54,-0.035997415822383,1.34));
#35134=CARTESIAN_POINT('Origin',(0.,0.,1.34));
#35135=CARTESIAN_POINT('Origin',(-0.54,-0.035997415822383,0.66));
#35136=CARTESIAN_POINT('',(-0.499858037235396,-0.0119139670629816,0.66));
#35137=CARTESIAN_POINT('',(-0.499858037235396,-0.0119139670629816,1.));
#35138=CARTESIAN_POINT('',(-0.54,-0.035997415822383,0.66));
#35139=CARTESIAN_POINT('Origin',(-0.51,5.55111512312578E-17,0.66));
#35140=CARTESIAN_POINT('',(-0.5,-6.12323399573677E-17,0.66));
#35141=CARTESIAN_POINT('Origin',(0.,0.,0.66));
#35142=CARTESIAN_POINT('Origin',(0.,0.,0.66));
#35143=CARTESIAN_POINT('Origin',(-0.463644396618753,0.12423314164921,0.66));
#35144=CARTESIAN_POINT('',(-0.479742226065208,0.140880788363777,0.66));
#35145=CARTESIAN_POINT('',(-0.479742226065208,0.140880788363777,1.34));
#35146=CARTESIAN_POINT('',(-0.479742226065208,0.140880788363777,1.));
#35147=CARTESIAN_POINT('',(-0.463644396618753,0.12423314164921,0.66));
#35148=CARTESIAN_POINT('',(-0.463644396618753,0.12423314164921,0.66));
#35149=CARTESIAN_POINT('',(-0.463644396618753,0.12423314164921,1.34));
#35150=CARTESIAN_POINT('',(-0.463644396618753,0.12423314164921,0.66));
#35151=CARTESIAN_POINT('',(-0.463644396618753,0.12423314164921,1.34));
#35152=CARTESIAN_POINT('Origin',(-0.492622171407425,0.131997713002286,1.34));
#35153=CARTESIAN_POINT('',(-0.485909349222455,0.117864771404394,1.34));
#35154=CARTESIAN_POINT('Origin',(0.,0.,1.34));
#35155=CARTESIAN_POINT('',(-0.530916762985404,0.104991450732855,1.34));
#35156=CARTESIAN_POINT('Origin',(-0.530916762985404,0.104991450732855,0.66));
#35157=CARTESIAN_POINT('',(-0.485909349222455,0.117864771404394,0.66));
#35158=CARTESIAN_POINT('',(-0.485909349222455,0.117864771404394,1.));
#35159=CARTESIAN_POINT('',(-0.530916762985404,0.104991450732855,0.66));
#35160=CARTESIAN_POINT('Origin',(-0.492622171407425,0.131997713002286,0.66));
#35161=CARTESIAN_POINT('Origin',(0.,0.,0.66));
#35162=CARTESIAN_POINT('Origin',(-0.41569219381653,0.24,0.66));
#35163=CARTESIAN_POINT('',(-0.42693277500019,0.260246816754091,0.66));
#35164=CARTESIAN_POINT('',(-0.42693277500019,0.260246816754091,1.34));
#35165=CARTESIAN_POINT('',(-0.42693277500019,0.260246816754091,1.));
#35166=CARTESIAN_POINT('',(-0.41569219381653,0.24,0.66));
#35167=CARTESIAN_POINT('',(-0.41569219381653,0.24,0.66));
#35168=CARTESIAN_POINT('',(-0.41569219381653,0.24,1.34));
#35169=CARTESIAN_POINT('',(-0.41569219381653,0.24,0.66));
#35170=CARTESIAN_POINT('',(-0.41569219381653,0.24,1.34));
#35171=CARTESIAN_POINT('Origin',(-0.441672955930064,0.255,1.34));
#35172=CARTESIAN_POINT('',(-0.438846742063171,0.239611220481305,1.34));
#35173=CARTESIAN_POINT('Origin',(0.,0.,1.34));
#35174=CARTESIAN_POINT('',(-0.485652425954788,0.238825323427225,1.34));
#35175=CARTESIAN_POINT('Origin',(-0.485652425954788,0.238825323427225,0.66));
#35176=CARTESIAN_POINT('',(-0.438846742063171,0.239611220481305,0.66));
#35177=CARTESIAN_POINT('',(-0.438846742063171,0.239611220481305,1.));
#35178=CARTESIAN_POINT('',(-0.485652425954788,0.238825323427225,0.66));
#35179=CARTESIAN_POINT('Origin',(-0.441672955930064,0.255,0.66));
#35180=CARTESIAN_POINT('Origin',(0.,0.,0.66));
#35181=CARTESIAN_POINT('Origin',(-0.339411254969543,0.339411254969543,0.66));
#35182=CARTESIAN_POINT('',(-0.345028560858679,0.361877454660814,0.66));
#35183=CARTESIAN_POINT('',(-0.345028560858679,0.361877454660814,1.34));
#35184=CARTESIAN_POINT('',(-0.345028560858679,0.361877454660814,1.));
#35185=CARTESIAN_POINT('',(-0.339411254969543,0.339411254969543,0.66));
#35186=CARTESIAN_POINT('',(-0.339411254969543,0.339411254969543,0.66));
#35187=CARTESIAN_POINT('',(-0.339411254969543,0.339411254969543,1.34));
#35188=CARTESIAN_POINT('',(-0.339411254969543,0.339411254969543,0.66));
#35189=CARTESIAN_POINT('',(-0.339411254969543,0.339411254969543,1.34));
#35190=CARTESIAN_POINT('Origin',(-0.360624458405139,0.360624458405139,1.34));
#35191=CARTESIAN_POINT('',(-0.361877454660814,0.345028560858679,1.34));
#35192=CARTESIAN_POINT('Origin',(0.,0.,1.34));
#35193=CARTESIAN_POINT('',(-0.407291678673935,0.356383645007537,1.34));
#35194=CARTESIAN_POINT('Origin',(-0.407291678673935,0.356383645007537,0.66));
#35195=CARTESIAN_POINT('',(-0.361877454660814,0.345028560858679,0.66));
#35196=CARTESIAN_POINT('',(-0.361877454660814,0.345028560858679,1.));
#35197=CARTESIAN_POINT('',(-0.407291678673935,0.356383645007537,0.66));
#35198=CARTESIAN_POINT('Origin',(-0.360624458405139,0.360624458405139,0.66));
#35199=CARTESIAN_POINT('Origin',(0.,0.,0.66));
#35200=CARTESIAN_POINT('Origin',(-0.24,0.415692193816531,0.66));
#35201=CARTESIAN_POINT('',(-0.239611220481305,0.438846742063171,0.66));
#35202=CARTESIAN_POINT('',(-0.239611220481305,0.438846742063171,1.34));
#35203=CARTESIAN_POINT('',(-0.239611220481305,0.438846742063171,1.));
#35204=CARTESIAN_POINT('',(-0.24,0.415692193816531,0.66));
#35205=CARTESIAN_POINT('',(-0.24,0.415692193816531,0.66));
#35206=CARTESIAN_POINT('',(-0.24,0.415692193816531,1.34));
#35207=CARTESIAN_POINT('',(-0.24,0.415692193816531,0.66));
#35208=CARTESIAN_POINT('',(-0.24,0.415692193816531,1.34));
#35209=CARTESIAN_POINT('Origin',(-0.255,0.441672955930064,1.34));
#35210=CARTESIAN_POINT('',(-0.260246816754091,0.42693277500019,1.34));
#35211=CARTESIAN_POINT('Origin',(0.,0.,1.34));
#35212=CARTESIAN_POINT('',(-0.301174676572776,0.449655010132405,1.34));
#35213=CARTESIAN_POINT('Origin',(-0.301174676572776,0.449655010132405,0.66));
#35214=CARTESIAN_POINT('',(-0.260246816754091,0.42693277500019,0.66));
#35215=CARTESIAN_POINT('',(-0.260246816754091,0.42693277500019,1.));
#35216=CARTESIAN_POINT('',(-0.301174676572776,0.449655010132405,0.66));
#35217=CARTESIAN_POINT('Origin',(-0.255,0.441672955930064,0.66));
#35218=CARTESIAN_POINT('Origin',(0.,0.,0.66));
#35219=CARTESIAN_POINT('Origin',(-0.12423314164921,0.463644396618753,0.66));
#35220=CARTESIAN_POINT('',(-0.117864771404394,0.485909349222455,0.66));
#35221=CARTESIAN_POINT('',(-0.117864771404394,0.485909349222455,1.34));
#35222=CARTESIAN_POINT('',(-0.117864771404394,0.485909349222455,1.));
#35223=CARTESIAN_POINT('',(-0.12423314164921,0.463644396618753,0.66));
#35224=CARTESIAN_POINT('',(-0.12423314164921,0.463644396618753,0.66));
#35225=CARTESIAN_POINT('',(-0.12423314164921,0.463644396618753,1.34));
#35226=CARTESIAN_POINT('',(-0.12423314164921,0.463644396618753,0.66));
#35227=CARTESIAN_POINT('',(-0.12423314164921,0.463644396618753,1.34));
#35228=CARTESIAN_POINT('Origin',(-0.131997713002286,0.492622171407425,1.34));
#35229=CARTESIAN_POINT('',(-0.140880788363777,0.479742226065208,1.34));
#35230=CARTESIAN_POINT('Origin',(0.,0.,1.34));
#35231=CARTESIAN_POINT('',(-0.174533117977868,0.512283129406789,1.34));
#35232=CARTESIAN_POINT('Origin',(-0.174533117977868,0.512283129406789,0.66));
#35233=CARTESIAN_POINT('',(-0.140880788363777,0.479742226065208,0.66));
#35234=CARTESIAN_POINT('',(-0.140880788363777,0.479742226065208,1.));
#35235=CARTESIAN_POINT('',(-0.174533117977868,0.512283129406789,0.66));
#35236=CARTESIAN_POINT('Origin',(-0.131997713002286,0.492622171407425,0.66));
#35237=CARTESIAN_POINT('Origin',(0.,0.,0.66));
#35238=CARTESIAN_POINT('Origin',(2.77555756156289E-17,0.48,0.66));
#35239=CARTESIAN_POINT('',(0.0119139670629818,0.499858037235396,0.66));
#35240=CARTESIAN_POINT('',(0.0119139670629818,0.499858037235396,1.34));
#35241=CARTESIAN_POINT('',(0.0119139670629818,0.499858037235396,1.));
#35242=CARTESIAN_POINT('',(2.77555756156289E-17,0.48,0.66));
#35243=CARTESIAN_POINT('',(2.77555756156289E-17,0.48,0.66));
#35244=CARTESIAN_POINT('',(2.77555756156289E-17,0.48,1.34));
#35245=CARTESIAN_POINT('',(2.77555756156289E-17,0.48,0.66));
#35246=CARTESIAN_POINT('',(2.77555756156289E-17,0.48,1.34));
#35247=CARTESIAN_POINT('Origin',(2.77555756156289E-17,0.51,1.34));
#35248=CARTESIAN_POINT('',(-0.0119139670629817,0.499858037235396,1.34));
#35249=CARTESIAN_POINT('Origin',(0.,0.,1.34));
#35250=CARTESIAN_POINT('',(-0.035997415822383,0.54,1.34));
#35251=CARTESIAN_POINT('Origin',(-0.035997415822383,0.54,0.66));
#35252=CARTESIAN_POINT('',(-0.0119139670629817,0.499858037235396,0.66));
#35253=CARTESIAN_POINT('',(-0.0119139670629817,0.499858037235396,1.));
#35254=CARTESIAN_POINT('',(-0.035997415822383,0.54,0.66));
#35255=CARTESIAN_POINT('Origin',(2.77555756156289E-17,0.51,0.66));
#35256=CARTESIAN_POINT('Origin',(0.,0.,0.66));
#35257=CARTESIAN_POINT('Origin',(0.12423314164921,0.463644396618753,0.66));
#35258=CARTESIAN_POINT('',(0.140880788363777,0.479742226065208,0.66));
#35259=CARTESIAN_POINT('',(0.140880788363777,0.479742226065208,1.34));
#35260=CARTESIAN_POINT('',(0.140880788363777,0.479742226065208,1.));
#35261=CARTESIAN_POINT('',(0.12423314164921,0.463644396618753,0.66));
#35262=CARTESIAN_POINT('',(0.12423314164921,0.463644396618753,0.66));
#35263=CARTESIAN_POINT('',(0.12423314164921,0.463644396618753,1.34));
#35264=CARTESIAN_POINT('',(0.12423314164921,0.463644396618753,0.66));
#35265=CARTESIAN_POINT('',(0.12423314164921,0.463644396618753,1.34));
#35266=CARTESIAN_POINT('Origin',(0.131997713002286,0.492622171407425,1.34));
#35267=CARTESIAN_POINT('',(0.117864771404394,0.485909349222455,1.34));
#35268=CARTESIAN_POINT('Origin',(0.,0.,1.34));
#35269=CARTESIAN_POINT('',(0.104991450732855,0.530916762985404,1.34));
#35270=CARTESIAN_POINT('Origin',(0.104991450732855,0.530916762985404,0.66));
#35271=CARTESIAN_POINT('',(0.117864771404394,0.485909349222455,0.66));
#35272=CARTESIAN_POINT('',(0.117864771404394,0.485909349222455,1.));
#35273=CARTESIAN_POINT('',(0.104991450732855,0.530916762985404,0.66));
#35274=CARTESIAN_POINT('Origin',(0.131997713002286,0.492622171407425,0.66));
#35275=CARTESIAN_POINT('Origin',(0.,0.,0.66));
#35276=CARTESIAN_POINT('Origin',(0.24,0.415692193816531,0.66));
#35277=CARTESIAN_POINT('',(0.260246816754091,0.42693277500019,0.66));
#35278=CARTESIAN_POINT('',(0.260246816754091,0.42693277500019,1.34));
#35279=CARTESIAN_POINT('',(0.260246816754091,0.42693277500019,1.));
#35280=CARTESIAN_POINT('',(0.24,0.415692193816531,0.66));
#35281=CARTESIAN_POINT('',(0.24,0.415692193816531,0.66));
#35282=CARTESIAN_POINT('',(0.24,0.415692193816531,1.34));
#35283=CARTESIAN_POINT('',(0.24,0.415692193816531,0.66));
#35284=CARTESIAN_POINT('',(0.24,0.415692193816531,1.34));
#35285=CARTESIAN_POINT('Origin',(0.255,0.441672955930064,1.34));
#35286=CARTESIAN_POINT('',(0.239611220481305,0.438846742063171,1.34));
#35287=CARTESIAN_POINT('Origin',(0.,0.,1.34));
#35288=CARTESIAN_POINT('',(0.238825323427224,0.485652425954788,1.34));
#35289=CARTESIAN_POINT('Origin',(0.238825323427224,0.485652425954788,0.66));
#35290=CARTESIAN_POINT('',(0.239611220481305,0.438846742063171,0.66));
#35291=CARTESIAN_POINT('',(0.239611220481305,0.438846742063171,1.));
#35292=CARTESIAN_POINT('',(0.238825323427224,0.485652425954788,0.66));
#35293=CARTESIAN_POINT('Origin',(0.255,0.441672955930064,0.66));
#35294=CARTESIAN_POINT('Origin',(0.,0.,0.66));
#35295=CARTESIAN_POINT('Origin',(0.339411254969543,0.339411254969543,0.66));
#35296=CARTESIAN_POINT('',(0.361877454660814,0.345028560858679,0.66));
#35297=CARTESIAN_POINT('',(0.361877454660814,0.345028560858679,1.34));
#35298=CARTESIAN_POINT('',(0.361877454660814,0.345028560858679,1.));
#35299=CARTESIAN_POINT('',(0.339411254969543,0.339411254969543,0.66));
#35300=CARTESIAN_POINT('',(0.339411254969543,0.339411254969543,0.66));
#35301=CARTESIAN_POINT('',(0.339411254969543,0.339411254969543,1.34));
#35302=CARTESIAN_POINT('',(0.339411254969543,0.339411254969543,0.66));
#35303=CARTESIAN_POINT('',(0.339411254969543,0.339411254969543,1.34));
#35304=CARTESIAN_POINT('Origin',(0.360624458405139,0.360624458405139,1.34));
#35305=CARTESIAN_POINT('',(0.345028560858679,0.361877454660814,1.34));
#35306=CARTESIAN_POINT('Origin',(0.,0.,1.34));
#35307=CARTESIAN_POINT('',(0.356383645007537,0.407291678673935,1.34));
#35308=CARTESIAN_POINT('Origin',(0.356383645007537,0.407291678673935,0.66));
#35309=CARTESIAN_POINT('',(0.345028560858679,0.361877454660814,0.66));
#35310=CARTESIAN_POINT('',(0.345028560858679,0.361877454660814,1.));
#35311=CARTESIAN_POINT('',(0.356383645007537,0.407291678673935,0.66));
#35312=CARTESIAN_POINT('Origin',(0.360624458405139,0.360624458405139,0.66));
#35313=CARTESIAN_POINT('Origin',(0.,0.,0.66));
#35314=CARTESIAN_POINT('Origin',(0.415692193816531,0.24,0.66));
#35315=CARTESIAN_POINT('',(0.438846742063171,0.239611220481305,0.66));
#35316=CARTESIAN_POINT('',(0.438846742063171,0.239611220481305,1.34));
#35317=CARTESIAN_POINT('',(0.438846742063171,0.239611220481305,1.));
#35318=CARTESIAN_POINT('',(0.415692193816531,0.24,0.66));
#35319=CARTESIAN_POINT('',(0.415692193816531,0.24,0.66));
#35320=CARTESIAN_POINT('',(0.415692193816531,0.24,1.34));
#35321=CARTESIAN_POINT('',(0.415692193816531,0.24,0.66));
#35322=CARTESIAN_POINT('',(0.415692193816531,0.24,1.34));
#35323=CARTESIAN_POINT('Origin',(0.441672955930064,0.255,1.34));
#35324=CARTESIAN_POINT('',(0.42693277500019,0.260246816754091,1.34));
#35325=CARTESIAN_POINT('Origin',(0.,0.,1.34));
#35326=CARTESIAN_POINT('',(0.449655010132405,0.301174676572776,1.34));
#35327=CARTESIAN_POINT('Origin',(0.449655010132405,0.301174676572776,0.66));
#35328=CARTESIAN_POINT('',(0.42693277500019,0.260246816754091,0.66));
#35329=CARTESIAN_POINT('',(0.42693277500019,0.260246816754091,1.));
#35330=CARTESIAN_POINT('',(0.449655010132405,0.301174676572776,0.66));
#35331=CARTESIAN_POINT('Origin',(0.441672955930064,0.255,0.66));
#35332=CARTESIAN_POINT('Origin',(0.,0.,0.66));
#35333=CARTESIAN_POINT('Origin',(0.463644396618753,0.12423314164921,0.66));
#35334=CARTESIAN_POINT('',(0.485909349222455,0.117864771404394,0.66));
#35335=CARTESIAN_POINT('',(0.485909349222455,0.117864771404394,1.34));
#35336=CARTESIAN_POINT('',(0.485909349222455,0.117864771404394,1.));
#35337=CARTESIAN_POINT('',(0.463644396618753,0.12423314164921,0.66));
#35338=CARTESIAN_POINT('',(0.463644396618753,0.12423314164921,0.66));
#35339=CARTESIAN_POINT('',(0.463644396618753,0.12423314164921,1.34));
#35340=CARTESIAN_POINT('',(0.463644396618753,0.12423314164921,0.66));
#35341=CARTESIAN_POINT('',(0.463644396618753,0.12423314164921,1.34));
#35342=CARTESIAN_POINT('Origin',(0.492622171407425,0.131997713002286,1.34));
#35343=CARTESIAN_POINT('',(0.479742226065208,0.140880788363777,1.34));
#35344=CARTESIAN_POINT('Origin',(0.,0.,1.34));
#35345=CARTESIAN_POINT('',(0.512283129406789,0.174533117977868,1.34));
#35346=CARTESIAN_POINT('Origin',(0.512283129406789,0.174533117977868,0.66));
#35347=CARTESIAN_POINT('',(0.479742226065208,0.140880788363777,0.66));
#35348=CARTESIAN_POINT('',(0.479742226065208,0.140880788363777,1.));
#35349=CARTESIAN_POINT('',(0.512283129406789,0.174533117977868,0.66));
#35350=CARTESIAN_POINT('Origin',(0.492622171407425,0.131997713002286,0.66));
#35351=CARTESIAN_POINT('Origin',(0.,0.,0.66));
#35352=CARTESIAN_POINT('Origin',(0.48,0.,0.66));
#35353=CARTESIAN_POINT('',(0.499858037235396,-0.0119139670629817,0.66));
#35354=CARTESIAN_POINT('',(0.499858037235396,-0.0119139670629817,1.34));
#35355=CARTESIAN_POINT('',(0.499858037235396,-0.0119139670629817,1.));
#35356=CARTESIAN_POINT('',(0.48,0.,0.66));
#35357=CARTESIAN_POINT('',(0.48,0.,0.66));
#35358=CARTESIAN_POINT('',(0.48,0.,1.34));
#35359=CARTESIAN_POINT('',(0.48,0.,0.66));
#35360=CARTESIAN_POINT('',(0.48,0.,1.34));
#35361=CARTESIAN_POINT('Origin',(0.51,0.,1.34));
#35362=CARTESIAN_POINT('',(0.499858037235396,0.0119139670629817,1.34));
#35363=CARTESIAN_POINT('Origin',(0.,0.,1.34));
#35364=CARTESIAN_POINT('',(0.54,0.035997415822383,1.34));
#35365=CARTESIAN_POINT('Origin',(0.54,0.035997415822383,0.66));
#35366=CARTESIAN_POINT('',(0.499858037235396,0.0119139670629817,0.66));
#35367=CARTESIAN_POINT('',(0.499858037235396,0.0119139670629817,1.));
#35368=CARTESIAN_POINT('',(0.54,0.035997415822383,0.66));
#35369=CARTESIAN_POINT('Origin',(0.51,0.,0.66));
#35370=CARTESIAN_POINT('Origin',(0.,0.,0.66));
#35371=CARTESIAN_POINT('Origin',(0.,0.,1.43));
#35372=CARTESIAN_POINT('',(-0.06,-7.34788079488412E-18,1.66));
#35373=CARTESIAN_POINT('Origin',(0.,0.,1.66));
#35374=CARTESIAN_POINT('',(-0.06,-7.34788079488412E-18,1.2));
#35375=CARTESIAN_POINT('',(-0.06,-7.34788079488412E-18,1.43));
#35376=CARTESIAN_POINT('Origin',(0.,0.,1.2));
#35377=CARTESIAN_POINT('Origin',(0.,0.,1.68));
#35378=CARTESIAN_POINT('',(-0.0300000000000001,-3.67394039744207E-18,1.7));
#35379=CARTESIAN_POINT('Origin',(0.,0.,1.7));
#35380=CARTESIAN_POINT('',(-0.045,-5.51091059616309E-18,1.68));
#35381=CARTESIAN_POINT('Origin',(0.,0.,1.7));
#35382=CARTESIAN_POINT('Origin',(0.25,0.,1.2));
#35383=CARTESIAN_POINT('',(-0.25,-3.06161699786838E-17,1.2));
#35384=CARTESIAN_POINT('Origin',(0.,0.,1.2));
#35385=CARTESIAN_POINT('Origin',(0.,0.,1.525));
#35386=CARTESIAN_POINT('',(-0.25,3.06161699786838E-17,1.8));
#35387=CARTESIAN_POINT('',(-0.25,-3.06161699786838E-17,1.525));
#35388=CARTESIAN_POINT('Origin',(0.,0.,1.8));
#35389=CARTESIAN_POINT('Origin',(0.,0.,1.));
#35390=CARTESIAN_POINT('',(-0.5,-6.12323399573677E-17,1.4));
#35391=CARTESIAN_POINT('Origin',(0.,0.,1.4));
#35392=CARTESIAN_POINT('',(-0.5,-6.12323399573677E-17,1.));
#35393=CARTESIAN_POINT('',(-0.5,-6.12323399573677E-17,0.6));
#35394=CARTESIAN_POINT('',(-0.5,-6.12323399573677E-17,1.));
#35395=CARTESIAN_POINT('Origin',(0.,0.,0.6));
#35396=CARTESIAN_POINT('Origin',(0.52,0.,1.4));
#35397=CARTESIAN_POINT('',(-0.52,-6.36816335556624E-17,1.4));
#35398=CARTESIAN_POINT('Origin',(0.,0.,1.4));
#35399=CARTESIAN_POINT('Origin',(0.,0.,1.58));
#35400=CARTESIAN_POINT('',(-0.52,-6.36816335556624E-17,1.76));
#35401=CARTESIAN_POINT('Origin',(0.,0.,1.76));
#35402=CARTESIAN_POINT('',(-0.52,-6.36816335556624E-17,1.58));
#35403=CARTESIAN_POINT('Origin',(0.,0.,1.78));
#35404=CARTESIAN_POINT('',(-0.48,-5.8783046359073E-17,1.8));
#35405=CARTESIAN_POINT('Origin',(0.,0.,1.8));
#35406=CARTESIAN_POINT('',(-0.5,-6.12323399573677E-17,1.78));
#35407=CARTESIAN_POINT('Origin',(0.,0.,1.8));
#35408=CARTESIAN_POINT('Origin',(-0.317542648054294,-0.55,0.2));
#35409=CARTESIAN_POINT('',(0.317542648054294,-0.55,0.2));
#35410=CARTESIAN_POINT('',(-0.317542648054294,-0.55,0.2));
#35411=CARTESIAN_POINT('',(-0.158771324027147,-0.55,0.2));
#35412=CARTESIAN_POINT('',(0.317542648054294,-0.55,0.6));
#35413=CARTESIAN_POINT('',(0.317542648054294,-0.55,0.2));
#35414=CARTESIAN_POINT('',(-0.317542648054294,-0.55,0.6));
#35415=CARTESIAN_POINT('',(-0.317542648054294,-0.55,0.6));
#35416=CARTESIAN_POINT('',(-0.317542648054294,-0.55,0.2));
#35417=CARTESIAN_POINT('Origin',(-0.635085296108588,7.77755175064932E-17,
0.2));
#35418=CARTESIAN_POINT('',(-0.635085296108588,7.77755175064932E-17,0.2));
#35419=CARTESIAN_POINT('',(-0.555699634095015,-0.1375,0.2));
#35420=CARTESIAN_POINT('',(-0.635085296108588,1.11022302462516E-16,0.6));
#35421=CARTESIAN_POINT('',(-0.635085296108588,7.77755175064932E-17,0.6));
#35422=CARTESIAN_POINT('',(-0.635085296108588,7.77755175064932E-17,0.2));
#35423=CARTESIAN_POINT('Origin',(-0.317542648054294,0.55,0.2));
#35424=CARTESIAN_POINT('',(-0.317542648054294,0.55,0.2));
#35425=CARTESIAN_POINT('',(-0.396928310067868,0.4125,0.2));
#35426=CARTESIAN_POINT('',(-0.317542648054294,0.55,0.6));
#35427=CARTESIAN_POINT('',(-0.317542648054294,0.55,0.6));
#35428=CARTESIAN_POINT('',(-0.317542648054294,0.55,0.2));
#35429=CARTESIAN_POINT('Origin',(0.317542648054294,0.55,0.2));
#35430=CARTESIAN_POINT('',(0.317542648054294,0.55,0.2));
#35431=CARTESIAN_POINT('',(0.158771324027147,0.55,0.2));
#35432=CARTESIAN_POINT('',(0.317542648054294,0.55,0.6));
#35433=CARTESIAN_POINT('',(0.317542648054294,0.55,0.6));
#35434=CARTESIAN_POINT('',(0.317542648054294,0.55,0.2));
#35435=CARTESIAN_POINT('Origin',(0.635085296108588,0.,0.2));
#35436=CARTESIAN_POINT('',(0.635085296108588,0.,0.2));
#35437=CARTESIAN_POINT('',(0.555699634095015,0.1375,0.2));
#35438=CARTESIAN_POINT('',(0.635085296108588,0.,0.6));
#35439=CARTESIAN_POINT('',(0.635085296108588,0.,0.6));
#35440=CARTESIAN_POINT('',(0.635085296108588,0.,0.2));
#35441=CARTESIAN_POINT('Origin',(0.317542648054294,-0.55,0.2));
#35442=CARTESIAN_POINT('',(0.396928310067868,-0.4125,0.2));
#35443=CARTESIAN_POINT('',(0.317542648054294,-0.55,0.6));
#35444=CARTESIAN_POINT('Origin',(0.,1.11022302462516E-16,0.6));
#35445=CARTESIAN_POINT('Origin',(0.,0.,0.));
#35446=CARTESIAN_POINT('',(-0.7,0.7,0.));
#35447=CARTESIAN_POINT('',(-0.7,-0.7,0.));
#35448=CARTESIAN_POINT('',(-0.7,0.7,0.));
#35449=CARTESIAN_POINT('',(0.7,0.7,0.));
#35450=CARTESIAN_POINT('',(0.7,0.7,0.));
#35451=CARTESIAN_POINT('',(0.7,-0.7,0.));
#35452=CARTESIAN_POINT('',(0.7,-0.7,0.));
#35453=CARTESIAN_POINT('',(-0.7,-0.7,0.));
#35454=CARTESIAN_POINT('Origin',(0.,0.,0.));
#35455=CARTESIAN_POINT('Origin',(0.7,0.7,0.));
#35456=CARTESIAN_POINT('',(-0.7,0.7,0.2));
#35457=CARTESIAN_POINT('',(-0.7,0.7,0.));
#35458=CARTESIAN_POINT('',(0.7,0.7,0.2));
#35459=CARTESIAN_POINT('',(0.7,0.7,0.2));
#35460=CARTESIAN_POINT('',(0.7,0.7,0.));
#35461=CARTESIAN_POINT('Origin',(0.7,-0.7,0.));
#35462=CARTESIAN_POINT('',(0.7,-0.7,0.2));
#35463=CARTESIAN_POINT('',(0.7,-0.7,0.2));
#35464=CARTESIAN_POINT('',(0.7,-0.7,0.));
#35465=CARTESIAN_POINT('Origin',(-0.7,-0.7,0.));
#35466=CARTESIAN_POINT('',(-0.7,-0.7,0.2));
#35467=CARTESIAN_POINT('',(-0.7,-0.7,0.2));
#35468=CARTESIAN_POINT('',(-0.7,-0.7,0.));
#35469=CARTESIAN_POINT('Origin',(-0.7,0.7,0.));
#35470=CARTESIAN_POINT('',(-0.7,0.7,0.2));
#35471=CARTESIAN_POINT('Origin',(0.,0.,0.2));
#35472=CARTESIAN_POINT('Origin',(0.36,0.,-1.));
#35473=CARTESIAN_POINT('',(-0.36,-4.40872847693047E-17,-1.));
#35474=CARTESIAN_POINT('Origin',(0.,0.,-1.));
#35475=CARTESIAN_POINT('Origin',(0.,0.,-0.98));
#35476=CARTESIAN_POINT('',(-0.38,-4.65365783675994E-17,-0.98));
#35477=CARTESIAN_POINT('Origin',(0.,0.,-0.48));
#53621=UNCERTAINTY_MEASURE_WITH_UNIT(LENGTH_MEASURE(0.001),#53651,
'DISTANCE_ACCURACY_VALUE',
'Maximum model space distance between geometric entities at asserted c
onnectivities');
#53632=UNCERTAINTY_MEASURE_WITH_UNIT(LENGTH_MEASURE(0.001),#53651,
'DISTANCE_ACCURACY_VALUE',
'Maximum model space distance between geometric entities at asserted c
onnectivities');
#53639=(
GEOMETRIC_REPRESENTATION_CONTEXT(3)
GLOBAL_UNCERTAINTY_ASSIGNED_CONTEXT((#53621))
GLOBAL_UNIT_ASSIGNED_CONTEXT((#53651,#53653,#53654))
REPRESENTATION_CONTEXT('','3D')
);
#53650=(
GEOMETRIC_REPRESENTATION_CONTEXT(3)
GLOBAL_UNCERTAINTY_ASSIGNED_CONTEXT((#53632))
GLOBAL_UNIT_ASSIGNED_CONTEXT((#53651,#53653,#53654))
REPRESENTATION_CONTEXT('','3D')
);
#53651=(
LENGTH_UNIT()
NAMED_UNIT(*)
SI_UNIT(.CENTI.,.METRE.)
);
#53653=(
NAMED_UNIT(*)
PLANE_ANGLE_UNIT()
SI_UNIT($,.RADIAN.)
);
#53654=(
NAMED_UNIT(*)
SI_UNIT($,.STERADIAN.)
SOLID_ANGLE_UNIT()
);
#53661=SHAPE_DEFINITION_REPRESENTATION(#53678,#53729);
#53678=PRODUCT_DEFINITION_SHAPE('',$,#53747);
#53729=SHAPE_REPRESENTATION('',(#24107),#53639);
#53740=PRODUCT_DEFINITION_CONTEXT('part definition',#53793,'design');
#53747=PRODUCT_DEFINITION('2026-10-18-22-44-54-812',
'13_SHV_High-Voltage_Cable_Terminal_Plug',#53764,#53740);
#53764=PRODUCT_DEFINITION_FORMATION('',$,#53801);
#53793=APPLICATION_CONTEXT(
'Core Data for Automotive Mechanical Design Process');
#53794=PRODUCT_CONTEXT('part definition',#53793,'mechanical');
#53801=PRODUCT('2026-10-18-22-44-54-812',
'13_SHV_High-Voltage_Cable_Terminal_Plug',$,(#53794));
#53966=COLOUR_RGB('Off White',0.89,0.88,0.83);
#53967=FILL_AREA_STYLE_COLOUR('',#53966);
#53968=FILL_AREA_STYLE('',(#53967));
#53969=SURFACE_STYLE_FILL_AREA(#53968);
#53970=SURFACE_SIDE_STYLE('',(#53969));
#53971=SURFACE_STYLE_USAGE(.BOTH.,#53970);
#53972=PRESENTATION_STYLE_ASSIGNMENT((#53971));
ENDSEC;
END-ISO-10303-21;
